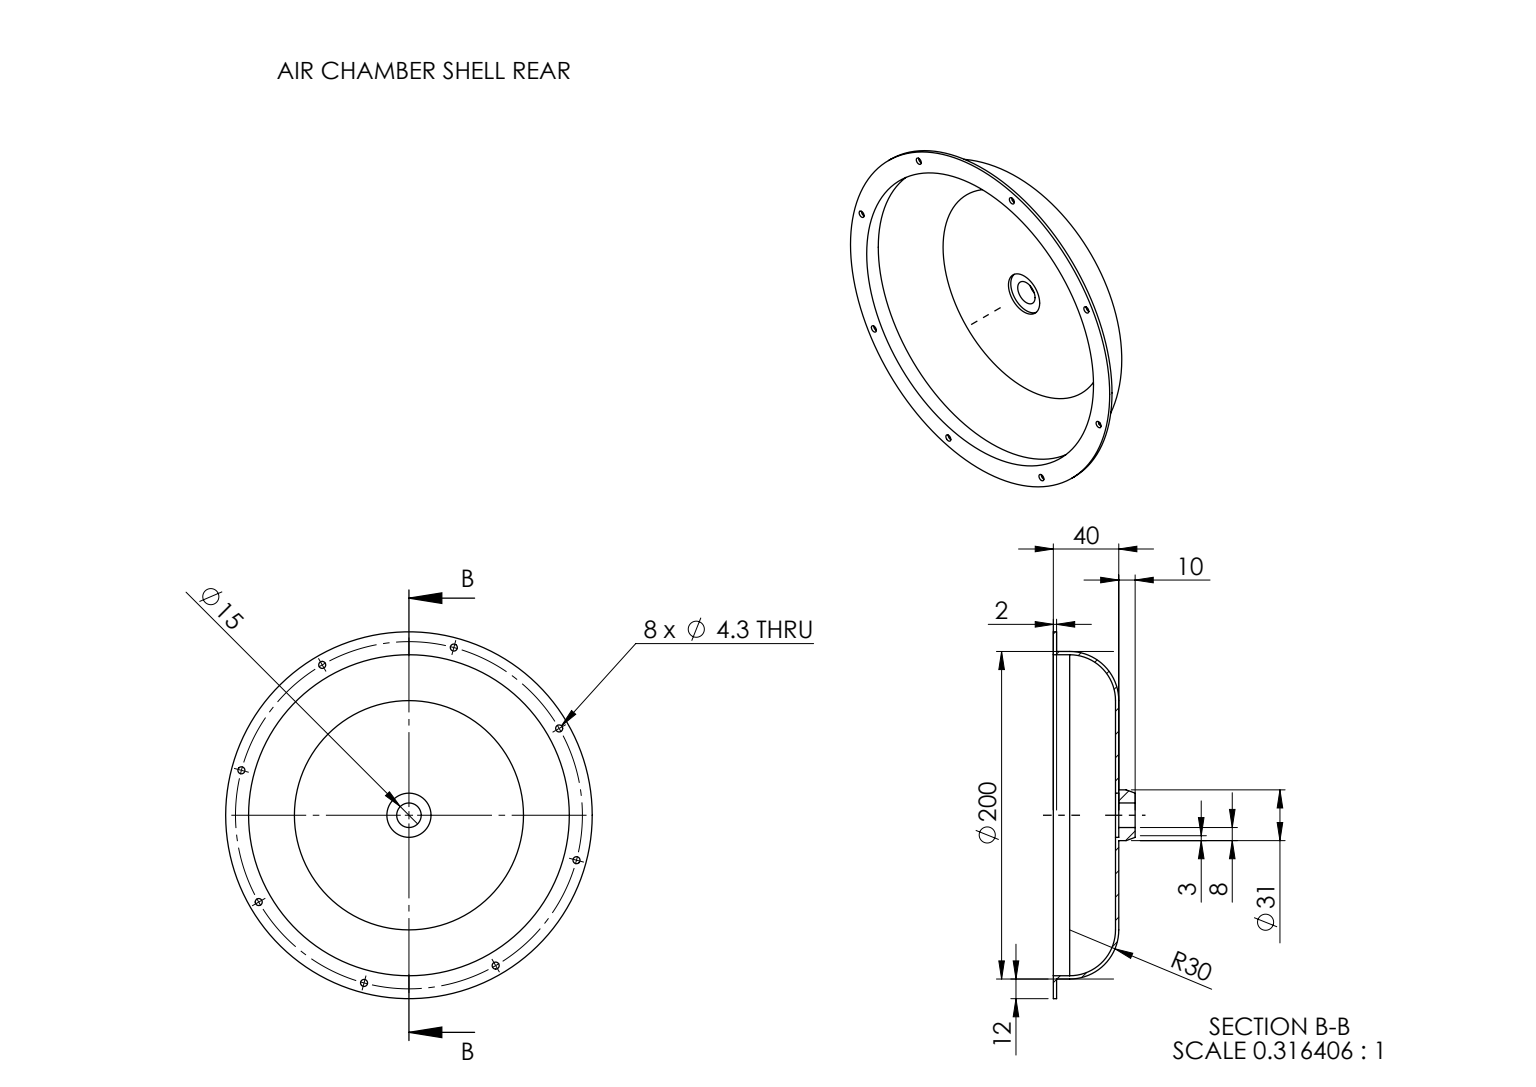
ISO-10303-21;
HEADER;
FILE_DESCRIPTION (('STEP AP214'),
    '1' );
FILE_NAME ('air chamber shell rear.step',
    '2026-10-08T07:58:12',
    ( '' ),
    ( '' ),
    'SwSTEP 2.0',
    'SolidWorks 2026',
    '' );
FILE_SCHEMA (( 'AUTOMOTIVE_DESIGN' ));
ENDSEC;

DATA;
#7=DIRECTION ( 'NONE',  ( 0.000000000000000000, 0.000000000000000000, -1.000000000000000000 ) ) ;
#68=ORIENTED_EDGE ( 'NONE', *, *, #26579, .F. ) ;
#75=AXIS2_PLACEMENT_3D ( 'NONE', #16121, #13402, #469 ) ;
#77=DIRECTION ( 'NONE',  ( -1.000000000000000000, -0.000000000000000000, -0.000000000000000000 ) ) ;
#93=PLANE ( 'NONE',  #4285 ) ;
#101=CIRCLE ( 'NONE', #26212, 13.50000000000001066 ) ;
#171=VERTEX_POINT ( 'NONE', #1955 ) ;
#187=CARTESIAN_POINT ( 'NONE',  ( 107.5000000000000000, 155.0000000000000000, -6.938893903907228378E-15 ) ) ;
#191=EDGE_CURVE ( 'NONE', #26009, #2264, #14724, .T. ) ;
#230=DIRECTION ( 'NONE',  ( 1.000000000000000000, 0.000000000000000000, 0.000000000000000000 ) ) ;
#283=ORIENTED_EDGE ( 'NONE', *, *, #23034, .T. ) ;
#304=CARTESIAN_POINT ( 'NONE',  ( 115.4999999999999858, 207.9999999999998010, -91.79869280115066488 ) ) ;
#307=FACE_BOUND ( 'NONE', #22866, .T. ) ;
#349=AXIS2_PLACEMENT_3D ( 'NONE', #10435, #20806, #13142 ) ;
#414=ORIENTED_EDGE ( 'NONE', *, *, #20724, .T. ) ;
#434=EDGE_CURVE ( 'NONE', #32282, #27762, #17038, .T. ) ;
#438=ORIENTED_EDGE ( 'NONE', *, *, #191, .T. ) ;
#454=ORIENTED_EDGE ( 'NONE', *, *, #17916, .T. ) ;
#462=SURFACE_STYLE_USAGE ( .BOTH. , #25511 ) ;
#469=DIRECTION ( 'NONE',  ( 0.000000000000000000, 0.000000000000000000, -1.000000000000000000 ) ) ;
#492=CONICAL_SURFACE ( 'NONE', #30975, 15.50000000000001066, 0.3490658503988691153 ) ;
#506=( LENGTH_UNIT ( ) NAMED_UNIT ( * ) SI_UNIT ( .MILLI., .METRE. ) );
#529=ORIENTED_EDGE ( 'NONE', *, *, #7683, .F. ) ;
#536=VERTEX_POINT ( 'NONE', #28106 ) ;
#540=ORIENTED_EDGE ( 'NONE', *, *, #17503, .F. ) ;
#598=EDGE_CURVE ( 'NONE', #2264, #27762, #4180, .T. ) ;
#600=CARTESIAN_POINT ( 'NONE',  ( 115.4999999999999858, 155.0000000000000000, -6.938893903907228378E-15 ) ) ;
#625=DIRECTION ( 'NONE',  ( 0.000000000000000000, 0.000000000000000000, -1.000000000000000000 ) ) ;
#670=PRODUCT_CONTEXT ( 'NONE', #3757, 'mechanical' ) ;
#673=CONICAL_SURFACE ( 'NONE', #14801, 15.50000000000001066, 0.3490658503988691153 ) ;
#713=FACE_OUTER_BOUND ( 'NONE', #1487, .T. ) ;
#776=CIRCLE ( 'NONE', #1871, 69.99999999999998579 ) ;
#832=SURFACE_STYLE_FILL_AREA ( #18565 ) ;
#833=DIRECTION ( 'NONE',  ( 0.000000000000000000, 0.000000000000000000, -1.000000000000000000 ) ) ;
#862=ORIENTED_EDGE ( 'NONE', *, *, #26257, .T. ) ;
#903=PRODUCT_DEFINITION_CONTEXT ( 'detailed design', #2680, 'design' ) ;
#950=CIRCLE ( 'NONE', #16649, 27.99999999999999645 ) ;
#961=CARTESIAN_POINT ( 'NONE',  ( 117.5000000000000000, 63.20130719884917170, -52.99999999999946709 ) ) ;
#971=AXIS2_PLACEMENT_3D ( 'NONE', #10766, #21306, #3410 ) ;
#1073=EDGE_LOOP ( 'NONE', ( #10094, #23123, #12443, #529 ) ) ;
#1133=FACE_OUTER_BOUND ( 'NONE', #17035, .T. ) ;
#1157=DIRECTION ( 'NONE',  ( 0.000000000000000000, 0.000000000000000000, -1.000000000000000000 ) ) ;
#1188=ORIENTED_EDGE ( 'NONE', *, *, #27275, .F. ) ;
#1230=CARTESIAN_POINT ( 'NONE',  ( 115.4999999999999858, 51.09158283380785548, 28.95509836041905771 ) ) ;
#1232=MANIFOLD_SOLID_BREP ( 'CirPattern1', #28098 ) ;
#1268=ORIENTED_EDGE ( 'NONE', *, *, #4948, .F. ) ;
#1283=ORIENTED_EDGE ( 'NONE', *, *, #598, .T. ) ;
#1365=EDGE_LOOP ( 'NONE', ( #22857, #1283 ) ) ;
#1371=EDGE_CURVE ( 'NONE', #3136, #6813, #17831, .T. ) ;
#1414=DIRECTION ( 'NONE',  ( 0.000000000000000000, 0.000000000000000000, -1.000000000000000000 ) ) ;
#1450=EDGE_LOOP ( 'NONE', ( #15818, #25203 ) ) ;
#1487=EDGE_LOOP ( 'NONE', ( #7285, #14189, #23041, #24412 ) ) ;
#1501=DIRECTION ( 'NONE',  ( 0.000000000000000000, 1.000000000000000000, -9.682177540335733218E-15 ) ) ;
#1530=CIRCLE ( 'NONE', #18391, 112.0000000000000426 ) ;
#1665=DIRECTION ( 'NONE',  ( 1.000000000000000000, 0.000000000000000000, 0.000000000000000000 ) ) ;
#1738=EDGE_LOOP ( 'NONE', ( #5719, #22132, #19511, #15323 ) ) ;
#1752=DIRECTION ( 'NONE',  ( 0.000000000000000000, -0.7071067811865434649, 0.7071067811865515695 ) ) ;
#1760=DIRECTION ( 'NONE',  ( -1.000000000000000000, 0.000000000000000000, -0.000000000000000000 ) ) ;
#1788=AXIS2_PLACEMENT_3D ( 'NONE', #23905, #3451, #6004 ) ;
#1798=ADVANCED_FACE ( 'NONE', ( #23430, #1969 ), #93, .T. ) ;
#1801=CARTESIAN_POINT ( 'NONE',  ( 117.5000000000000000, 61.05130719884917312, -52.99999999999945999 ) ) ;
#1817=CIRCLE ( 'NONE', #3443, 69.99999999999998579 ) ;
#1831=CARTESIAN_POINT ( 'NONE',  ( 115.4999999999999858, 102.0000000000001990, 91.79869280115065067 ) ) ;
#1852=DIRECTION ( 'NONE',  ( 1.000000000000000000, 0.000000000000000000, 0.000000000000000000 ) ) ;
#1862=ORIENTED_EDGE ( 'NONE', *, *, #7924, .F. ) ;
#1871=AXIS2_PLACEMENT_3D ( 'NONE', #22106, #6777, #17162 ) ;
#1916=VERTEX_POINT ( 'NONE', #11603 ) ;
#1943=DIRECTION ( 'NONE',  ( 0.000000000000000000, 0.000000000000000000, -1.000000000000000000 ) ) ;
#1955=CARTESIAN_POINT ( 'NONE',  ( 77.50000000000000000, 155.0000000000000000, -15.50000000000001776 ) ) ;
#1969=FACE_OUTER_BOUND ( 'NONE', #1365, .T. ) ;
#1973=VECTOR ( 'NONE', #1760, 1000.000000000000000 ) ;
#2026=AXIS2_PLACEMENT_3D ( 'NONE', #600, #24260, #8937 ) ;
#2045=VERTEX_POINT ( 'NONE', #8540 ) ;
#2054=ORIENTED_EDGE ( 'NONE', *, *, #8945, .T. ) ;
#2077=EDGE_LOOP ( 'NONE', ( #31532, #20694 ) ) ;
#2145=DIRECTION ( 'NONE',  ( -1.000000000000000000, 0.000000000000000000, 0.000000000000000000 ) ) ;
#2183=CYLINDRICAL_SURFACE ( 'NONE', #10236, 2.149999999999996803 ) ;
#2198=FACE_BOUND ( 'NONE', #2251, .T. ) ;
#2234=DIRECTION ( 'NONE',  ( 0.000000000000000000, 0.000000000000000000, -1.000000000000000000 ) ) ;
#2251=EDGE_LOOP ( 'NONE', ( #26956, #17710 ) ) ;
#2264=VERTEX_POINT ( 'NONE', #4435 ) ;
#2283=DIRECTION ( 'NONE',  ( 0.000000000000000000, -0.7071067811865540120, -0.7071067811865411334 ) ) ;
#2287=EDGE_CURVE ( 'NONE', #30017, #18599, #30683, .T. ) ;
#2336=CARTESIAN_POINT ( 'NONE',  ( 115.4999999999999858, 207.9999999999998010, -91.79869280115066488 ) ) ;
#2340=CIRCLE ( 'NONE', #6134, 98.00000000000000000 ) ;
#2351=EDGE_LOOP ( 'NONE', ( #6560, #11998 ) ) ;
#2383=AXIS2_PLACEMENT_3D ( 'NONE', #5252, #30654, #20597 ) ;
#2385=ORIENTED_EDGE ( 'NONE', *, *, #25125, .T. ) ;
#2404=AXIS2_PLACEMENT_3D ( 'NONE', #8872, #11941, #4266 ) ;
#2451=DIRECTION ( 'NONE',  ( 0.000000000000000000, 0.7071067811865475727, 0.7071067811865475727 ) ) ;
#2472=ORIENTED_EDGE ( 'NONE', *, *, #5437, .T. ) ;
#2481=CYLINDRICAL_SURFACE ( 'NONE', #11610, 2.149999999999999023 ) ;
#2516=ADVANCED_FACE ( 'NONE', ( #25896 ), #18566, .F. ) ;
#2537=FACE_BOUND ( 'NONE', #23999, .T. ) ;
#2601=FACE_OUTER_BOUND ( 'NONE', #15989, .T. ) ;
#2624=EDGE_CURVE ( 'NONE', #33027, #13306, #29875, .T. ) ;
#2637=DIRECTION ( 'NONE',  ( -1.000000000000000000, 0.000000000000000000, 0.000000000000000000 ) ) ;
#2680=APPLICATION_CONTEXT ( 'automotive_design' ) ;
#2681=AXIS2_PLACEMENT_3D ( 'NONE', #20295, #24901, #6678 ) ;
#2686=DIRECTION ( 'NONE',  ( -1.000000000000000000, -0.000000000000000000, -0.000000000000000000 ) ) ;
#2733=ORIENTED_EDGE ( 'NONE', *, *, #21234, .T. ) ;
#2774=AXIS2_PLACEMENT_3D ( 'NONE', #31193, #5458, #4959 ) ;
#2784=CARTESIAN_POINT ( 'NONE',  ( 79.50000000000000000, 155.0000000000000000, -69.99999999999998579 ) ) ;
#2786=FACE_BOUND ( 'NONE', #10971, .T. ) ;
#2808=ADVANCED_FACE ( 'NONE', ( #9001 ), #25061, .T. ) ;
#2811=EDGE_LOOP ( 'NONE', ( #20272, #1188, #20856, #9872 ) ) ;
#2863=CARTESIAN_POINT ( 'NONE',  ( 72.99495483890930814, 155.0000000000000000, -15.50000000000001776 ) ) ;
#2891=TOROIDAL_SURFACE ( 'NONE', #19225, 69.99999999999998579, 27.99999999999999645 ) ;
#2907=LINE ( 'NONE', #21126, #5343 ) ;
#2914=CARTESIAN_POINT ( 'NONE',  ( 115.4999999999999858, 51.09158283380784837, 28.95509836041906482 ) ) ;
#2953=CIRCLE ( 'NONE', #13273, 2.149999999999999023 ) ;
#3007=ORIENTED_EDGE ( 'NONE', *, *, #21235, .T. ) ;
#3010=DIRECTION ( 'NONE',  ( -1.000000000000000000, -0.000000000000000000, -0.000000000000000000 ) ) ;
#3081=EDGE_LOOP ( 'NONE', ( #11713, #8377, #3706, #13143 ) ) ;
#3082=EDGE_CURVE ( 'NONE', #10769, #27181, #18017, .T. ) ;
#3128=AXIS2_PLACEMENT_3D ( 'NONE', #20706, #25988, #29042 ) ;
#3136=VERTEX_POINT ( 'NONE', #33006 ) ;
#3150=DIRECTION ( 'NONE',  ( 1.000000000000000000, -0.000000000000000000, -0.000000000000000000 ) ) ;
#3162=AXIS2_PLACEMENT_3D ( 'NONE', #6462, #4579, #19574 ) ;
#3166=ORIENTED_EDGE ( 'NONE', *, *, #26579, .T. ) ;
#3182=AXIS2_PLACEMENT_3D ( 'NONE', #6530, #30205, #32410 ) ;
#3227=CARTESIAN_POINT ( 'NONE',  ( 115.4999999999999858, 126.0449016395812691, -103.9084171661922369 ) ) ;
#3230=VECTOR ( 'NONE', #6116, 1000.000000000000000 ) ;
#3252=EDGE_CURVE ( 'NONE', #5646, #15657, #33360, .T. ) ;
#3280=DIRECTION ( 'NONE',  ( -1.000000000000000000, 0.000000000000000000, -0.000000000000000000 ) ) ;
#3299=FACE_OUTER_BOUND ( 'NONE', #22987, .T. ) ;
#3328=EDGE_LOOP ( 'NONE', ( #4132, #17295 ) ) ;
#3354=ADVANCED_FACE ( 'NONE', ( #10372 ), #10201, .F. ) ;
#3410=DIRECTION ( 'NONE',  ( 0.000000000000000000, 0.000000000000000000, -1.000000000000000000 ) ) ;
#3433=CARTESIAN_POINT ( 'NONE',  ( 117.5000000000000000, 155.0000000000000000, -6.938893903907228378E-15 ) ) ;
#3443=AXIS2_PLACEMENT_3D ( 'NONE', #27976, #32741, #17244 ) ;
#3451=DIRECTION ( 'NONE',  ( 1.000000000000000000, 0.000000000000000000, 0.000000000000000000 ) ) ;
#3478=ORIENTED_EDGE ( 'NONE', *, *, #28138, .F. ) ;
#3558=SHAPE_DEFINITION_REPRESENTATION ( #12711, #19592 ) ;
#3599=CIRCLE ( 'NONE', #21614, 97.99999999999997158 ) ;
#3706=ORIENTED_EDGE ( 'NONE', *, *, #7107, .T. ) ;
#3709=EDGE_CURVE ( 'NONE', #5646, #31059, #20736, .T. ) ;
#3737=EDGE_CURVE ( 'NONE', #7925, #10430, #29432, .T. ) ;
#3757=APPLICATION_CONTEXT ( 'automotive_design' ) ;
#3823=VERTEX_POINT ( 'NONE', #30731 ) ;
#3850=CARTESIAN_POINT ( 'NONE',  ( 77.50000000000000000, 155.0000000000000000, -6.938893903907228378E-15 ) ) ;
#3894=EDGE_CURVE ( 'NONE', #10681, #3823, #25105, .T. ) ;
#3937=CARTESIAN_POINT ( 'NONE',  ( 115.4999999999999858, 155.0000000000000000, -6.938893903907228378E-15 ) ) ;
#3983=AXIS2_PLACEMENT_3D ( 'NONE', #32618, #27001, #19510 ) ;
#3984=CARTESIAN_POINT ( 'NONE',  ( 107.5000000000000000, 155.0000000000000000, 69.99999999999998579 ) ) ;
#4000=DIRECTION ( 'NONE',  ( 0.000000000000000000, -0.7071067811865346942, 0.7071067811865604513 ) ) ;
#4008=TOROIDAL_SURFACE ( 'NONE', #10009, 69.99999999999998579, 30.00000000000000000 ) ;
#4047=PLANE ( 'NONE',  #27123 ) ;
#4125=EDGE_LOOP ( 'NONE', ( #33172, #32411, #16064, #3478 ) ) ;
#4132=ORIENTED_EDGE ( 'NONE', *, *, #27275, .T. ) ;
#4180=CIRCLE ( 'NONE', #15058, 13.50000000000001066 ) ;
#4206=EDGE_LOOP ( 'NONE', ( #540, #18309 ) ) ;
#4221=AXIS2_PLACEMENT_3D ( 'NONE', #8999, #1665, #1501 ) ;
#4252=EDGE_CURVE ( 'NONE', #3823, #10681, #19124, .T. ) ;
#4266=DIRECTION ( 'NONE',  ( 1.000000000000000000, 0.000000000000000000, 0.000000000000000000 ) ) ;
#4285=AXIS2_PLACEMENT_3D ( 'NONE', #15423, #12866, #28550 ) ;
#4289=ORIENTED_EDGE ( 'NONE', *, *, #29372, .F. ) ;
#4300=CARTESIAN_POINT ( 'NONE',  ( 115.4999999999999858, 52.61186241335891367, 27.43481878086798176 ) ) ;
#4331=AXIS2_PLACEMENT_3D ( 'NONE', #18954, #26951, #10796 ) ;
#4332=ADVANCED_FACE ( 'NONE', ( #6323 ), #29500, .F. ) ;
#4349=VERTEX_POINT ( 'NONE', #27117 ) ;
#4352=CARTESIAN_POINT ( 'NONE',  ( 77.50000000000000000, 155.0000000000000000, 69.99999999999998579 ) ) ;
#4362=DIRECTION ( 'NONE',  ( 0.000000000000000000, 0.000000000000000000, 1.000000000000000000 ) ) ;
#4398=EDGE_CURVE ( 'NONE', #171, #13101, #11448, .T. ) ;
#4411=CARTESIAN_POINT ( 'NONE',  ( 115.4999999999999858, 244.6486928011512134, 52.99999999999884892 ) ) ;
#4426=EDGE_LOOP ( 'NONE', ( #26831, #11930, #30542, #23954 ) ) ;
#4435=CARTESIAN_POINT ( 'NONE',  ( 77.50000000000000000, 155.0000000000000000, -13.50000000000001776 ) ) ;
#4490=EDGE_CURVE ( 'NONE', #1916, #18599, #24575, .T. ) ;
#4499=LINE ( 'NONE', #28006, #21896 ) ;
#4514=CARTESIAN_POINT ( 'NONE',  ( 117.5000000000000000, 207.9999999999998010, -89.64869280115065919 ) ) ;
#4548=AXIS2_PLACEMENT_3D ( 'NONE', #31582, #8247, #11798 ) ;
#4566=ORIENTED_EDGE ( 'NONE', *, *, #8901, .F. ) ;
#4579=DIRECTION ( 'NONE',  ( 1.000000000000000000, 0.000000000000000000, 0.000000000000000000 ) ) ;
#4586=COLOUR_RGB ( '', 0.72549020, 0.75294118, 0.79215686) ;
#4604=CARTESIAN_POINT ( 'NONE',  ( 117.5000000000000000, 244.6486928011512134, 52.99999999999884892 ) ) ;
#4637=DIRECTION ( 'NONE',  ( 0.000000000000000000, 0.000000000000000000, -1.000000000000000000 ) ) ;
#4646=DIRECTION ( 'NONE',  ( 1.000000000000000000, 0.000000000000000000, 0.000000000000000000 ) ) ;
#4649=ORIENTED_EDGE ( 'NONE', *, *, #2624, .T. ) ;
#4688=CARTESIAN_POINT ( 'NONE',  ( 72.99495483890930814, 155.0000000000000000, -6.938893903907228378E-15 ) ) ;
#4690=CARTESIAN_POINT ( 'NONE',  ( 115.4999999999999858, 258.9084171661918958, -28.95509836041981444 ) ) ;
#4719=EDGE_CURVE ( 'NONE', #27181, #10769, #22400, .T. ) ;
#4762=ORIENTED_EDGE ( 'NONE', *, *, #17424, .T. ) ;
#4797=CIRCLE ( 'NONE', #3162, 112.0000000000000426 ) ;
#4802=ORIENTED_EDGE ( 'NONE', *, *, #598, .F. ) ;
#4822=DIRECTION ( 'NONE',  ( -1.000000000000000000, 0.000000000000000000, 0.000000000000000000 ) ) ;
#4862=LINE ( 'NONE', #28374, #29556 ) ;
#4902=ORIENTED_EDGE ( 'NONE', *, *, #19173, .F. ) ;
#4930=ORIENTED_EDGE ( 'NONE', *, *, #12672, .F. ) ;
#4948=EDGE_CURVE ( 'NONE', #22445, #13672, #13175, .T. ) ;
#4959=DIRECTION ( 'NONE',  ( 0.000000000000000000, 0.7071067811865442421, -0.7071067811865506814 ) ) ;
#4964=EDGE_CURVE ( 'NONE', #19918, #8949, #23184, .T. ) ;
#5016=ORIENTED_EDGE ( 'NONE', *, *, #29173, .F. ) ;
#5019=EDGE_CURVE ( 'NONE', #25798, #12782, #19635, .T. ) ;
#5023=EDGE_CURVE ( 'NONE', #18870, #7638, #28873, .T. ) ;
#5080=AXIS2_PLACEMENT_3D ( 'NONE', #23053, #4822, #22367 ) ;
#5102=ORIENTED_EDGE ( 'NONE', *, *, #28904, .T. ) ;
#5113=ORIENTED_EDGE ( 'NONE', *, *, #8496, .F. ) ;
#5136=ORIENTED_EDGE ( 'NONE', *, *, #19362, .F. ) ;
#5252=CARTESIAN_POINT ( 'NONE',  ( 117.5000000000000000, 127.5651812191323557, -102.3881375866411645 ) ) ;
#5279=CARTESIAN_POINT ( 'NONE',  ( 121.3406204335659879, 155.0000000000000000, -6.938893903907228378E-15 ) ) ;
#5303=DIRECTION ( 'NONE',  ( 0.9396926207859072067, 4.188538737677028743E-17, 0.3420201433256717105 ) ) ;
#5338=DIRECTION ( 'NONE',  ( -1.000000000000000000, 0.000000000000000000, 0.000000000000000000 ) ) ;
#5343=VECTOR ( 'NONE', #26085, 1000.000000000000000 ) ;
#5347=DIRECTION ( 'NONE',  ( -1.000000000000000000, -0.000000000000000000, 0.000000000000000000 ) ) ;
#5397=ORIENTED_EDGE ( 'NONE', *, *, #4252, .T. ) ;
#5437=EDGE_CURVE ( 'NONE', #10401, #5683, #4797, .T. ) ;
#5458=DIRECTION ( 'NONE',  ( -1.000000000000000000, 0.000000000000000000, 0.000000000000000000 ) ) ;
#5473=LINE ( 'NONE', #31537, #24283 ) ;
#5525=VECTOR ( 'NONE', #13656, 1000.000000000000000 ) ;
#5639=AXIS2_PLACEMENT_3D ( 'NONE', #31026, #25731, #28461 ) ;
#5646=VERTEX_POINT ( 'NONE', #4514 ) ;
#5670=DIRECTION ( 'NONE',  ( -1.000000000000000000, -0.000000000000000000, -0.000000000000000000 ) ) ;
#5683=VERTEX_POINT ( 'NONE', #22575 ) ;
#5719=ORIENTED_EDGE ( 'NONE', *, *, #3737, .F. ) ;
#5725=( NAMED_UNIT ( * ) PLANE_ANGLE_UNIT ( ) SI_UNIT ( $, .RADIAN. ) );
#5781=CARTESIAN_POINT ( 'NONE',  ( 79.50000000000000000, 155.0000000000000000, 13.50000000000000355 ) ) ;
#5787=DIRECTION ( 'NONE',  ( 0.000000000000000000, -1.000000000000000000, 9.682177540335733218E-15 ) ) ;
#5843=ORIENTED_EDGE ( 'NONE', *, *, #21234, .F. ) ;
#5862=DIRECTION ( 'NONE',  ( 0.000000000000000000, 1.000000000000000000, -3.227392513445223895E-15 ) ) ;
#5868=CYLINDRICAL_SURFACE ( 'NONE', #2026, 112.0000000000000426 ) ;
#5869=VERTEX_POINT ( 'NONE', #7927 ) ;
#5916=DIRECTION ( 'NONE',  ( 0.000000000000000000, -0.7071067811865540120, -0.7071067811865411334 ) ) ;
#5926=FACE_OUTER_BOUND ( 'NONE', #26057, .T. ) ;
#5953=EDGE_CURVE ( 'NONE', #21331, #2045, #25465, .T. ) ;
#5962=ORIENTED_EDGE ( 'NONE', *, *, #10995, .T. ) ;
#5965=ORIENTED_EDGE ( 'NONE', *, *, #20724, .F. ) ;
#6004=DIRECTION ( 'NONE',  ( 0.000000000000000000, 0.000000000000000000, -1.000000000000000000 ) ) ;
#6026=CARTESIAN_POINT ( 'NONE',  ( 115.4999999999999858, 63.20130719884917170, -52.99999999999946709 ) ) ;
#6031=EDGE_CURVE ( 'NONE', #20901, #28279, #1530, .T. ) ;
#6095=( NAMED_UNIT ( * ) PLANE_ANGLE_UNIT ( ) SI_UNIT ( $, .RADIAN. ) );
#6116=DIRECTION ( 'NONE',  ( -1.000000000000000000, 0.000000000000000000, 0.000000000000000000 ) ) ;
#6134=AXIS2_PLACEMENT_3D ( 'NONE', #9099, #7064, #25108 ) ;
#6139=AXIS2_PLACEMENT_3D ( 'NONE', #21230, #9074, #31625 ) ;
#6143=FACE_OUTER_BOUND ( 'NONE', #15317, .T. ) ;
#6154=DIRECTION ( 'NONE',  ( 0.000000000000000000, 0.000000000000000000, 1.000000000000000000 ) ) ;
#6178=AXIS2_PLACEMENT_3D ( 'NONE', #13035, #31270, #7931 ) ;
#6200=CYLINDRICAL_SURFACE ( 'NONE', #16792, 2.149999999999999023 ) ;
#6215=AXIS2_PLACEMENT_3D ( 'NONE', #31991, #19049, #29438 ) ;
#6217=ORIENTED_EDGE ( 'NONE', *, *, #19362, .T. ) ;
#6245=ADVANCED_FACE ( 'NONE', ( #22193 ), #32582, .F. ) ;
#6270=CARTESIAN_POINT ( 'NONE',  ( 117.5000000000000000, 127.5651812191323557, -102.3881375866411645 ) ) ;
#6319=CIRCLE ( 'NONE', #17271, 2.149999999999985256 ) ;
#6323=FACE_OUTER_BOUND ( 'NONE', #3081, .T. ) ;
#6365=DIRECTION ( 'NONE',  ( 0.000000000000000000, 0.000000000000000000, 1.000000000000000000 ) ) ;
#6462=CARTESIAN_POINT ( 'NONE',  ( 115.4999999999999858, 155.0000000000000000, -6.938893903907228378E-15 ) ) ;
#6530=CARTESIAN_POINT ( 'NONE',  ( 115.4999999999999858, 52.61186241335891367, 27.43481878086798176 ) ) ;
#6531=ORIENTED_EDGE ( 'NONE', *, *, #191, .F. ) ;
#6560=ORIENTED_EDGE ( 'NONE', *, *, #28904, .F. ) ;
#6567=ORIENTED_EDGE ( 'NONE', *, *, #17503, .T. ) ;
#6580=CARTESIAN_POINT ( 'NONE',  ( 77.50000000000000000, 155.0000000000000000, 15.50000000000000355 ) ) ;
#6592=ADVANCED_FACE ( 'NONE', ( #1133 ), #16798, .F. ) ;
#6621=AXIS2_PLACEMENT_3D ( 'NONE', #3433, #29167, #6154 ) ;
#6657=CARTESIAN_POINT ( 'NONE',  ( 115.4999999999999858, 102.0000000000001990, 89.64869280115064498 ) ) ;
#6678=DIRECTION ( 'NONE',  ( 0.000000000000000000, 0.000000000000000000, -1.000000000000000000 ) ) ;
#6770=MECHANICAL_DESIGN_GEOMETRIC_PRESENTATION_REPRESENTATION('',(#8929),#12761);
#6774=VERTEX_POINT ( 'NONE', #15086 ) ;
#6777=DIRECTION ( 'NONE',  ( -1.000000000000000000, -0.000000000000000000, -0.000000000000000000 ) ) ;
#6813=VERTEX_POINT ( 'NONE', #1801 ) ;
#6831=CYLINDRICAL_SURFACE ( 'NONE', #23613, 7.500000000000015099 ) ;
#6885=DIRECTION ( 'NONE',  ( 0.000000000000000000, 1.000000000000000000, -3.227392513445244800E-15 ) ) ;
#6892=CARTESIAN_POINT ( 'NONE',  ( 117.5000000000000000, 155.0000000000000000, -6.938893903907228378E-15 ) ) ;
#6902=VERTEX_POINT ( 'NONE', #28383 ) ;
#6919=CARTESIAN_POINT ( 'NONE',  ( 72.99495483890930814, 155.0000000000000000, -6.938893903907228378E-15 ) ) ;
#6935=DIRECTION ( 'NONE',  ( 0.000000000000000000, 0.000000000000000000, 1.000000000000000000 ) ) ;
#6984=ORIENTED_EDGE ( 'NONE', *, *, #27838, .F. ) ;
#7024=TOROIDAL_SURFACE ( 'NONE', #2681, 69.99999999999998579, 27.99999999999999645 ) ;
#7064=DIRECTION ( 'NONE',  ( 1.000000000000000000, 0.000000000000000000, 0.000000000000000000 ) ) ;
#7072=DIRECTION ( 'NONE',  ( -1.000000000000000000, -0.000000000000000000, -0.000000000000000000 ) ) ;
#7107=EDGE_CURVE ( 'NONE', #16763, #31655, #26322, .T. ) ;
#7142=DIRECTION ( 'NONE',  ( -1.000000000000000000, -0.000000000000000000, -0.000000000000000000 ) ) ;
#7145=AXIS2_PLACEMENT_3D ( 'NONE', #18693, #16919, #15797 ) ;
#7160=CARTESIAN_POINT ( 'NONE',  ( 77.50000000000000000, 155.0000000000000000, 13.50000000000000355 ) ) ;
#7166=AXIS2_PLACEMENT_3D ( 'NONE', #33449, #10120, #2451 ) ;
#7190=ADVANCED_FACE ( 'NONE', ( #21870 ), #6200, .F. ) ;
#7200=CIRCLE ( 'NONE', #20254, 2.149999999999999023 ) ;
#7254=ADVANCED_FACE ( 'NONE', ( #29711 ), #492, .T. ) ;
#7285=ORIENTED_EDGE ( 'NONE', *, *, #15353, .F. ) ;
#7302=CARTESIAN_POINT ( 'NONE',  ( 115.4999999999999858, 52.61186241335891367, 27.43481878086798176 ) ) ;
#7317=FACE_BOUND ( 'NONE', #15067, .T. ) ;
#7338=ORIENTED_EDGE ( 'NONE', *, *, #3709, .T. ) ;
#7340=DIRECTION ( 'NONE',  ( -1.000000000000000000, -0.000000000000000000, -0.000000000000000000 ) ) ;
#7406=LINE ( 'NONE', #12847, #17581 ) ;
#7427=ADVANCED_FACE ( 'NONE', ( #9782 ), #32429, .F. ) ;
#7451=ORIENTED_EDGE ( 'NONE', *, *, #20414, .T. ) ;
#7477=DIRECTION ( 'NONE',  ( 0.000000000000000000, 0.000000000000000000, 1.000000000000000000 ) ) ;
#7481=DIRECTION ( 'NONE',  ( 1.000000000000000000, 0.000000000000000000, 0.000000000000000000 ) ) ;
#7494=EDGE_CURVE ( 'NONE', #30420, #7638, #15710, .T. ) ;
#7540=ADVANCED_FACE ( 'NONE', ( #18123 ), #7738, .F. ) ;
#7545=EDGE_LOOP ( 'NONE', ( #22267, #16346 ) ) ;
#7557=CARTESIAN_POINT ( 'NONE',  ( 117.5000000000000000, 155.0000000000000000, -6.938893903907228378E-15 ) ) ;
#7571=CARTESIAN_POINT ( 'NONE',  ( 117.5000000000000000, 129.0854607986834424, -100.8678580070900921 ) ) ;
#7588=AXIS2_PLACEMENT_3D ( 'NONE', #21114, #33566, #28793 ) ;
#7638=VERTEX_POINT ( 'NONE', #12505 ) ;
#7683=EDGE_CURVE ( 'NONE', #3136, #27139, #31245, .T. ) ;
#7738=CYLINDRICAL_SURFACE ( 'NONE', #32579, 2.149999999999994138 ) ;
#7752=ORIENTED_EDGE ( 'NONE', *, *, #8496, .T. ) ;
#7814=FACE_OUTER_BOUND ( 'NONE', #8127, .T. ) ;
#7831=ORIENTED_EDGE ( 'NONE', *, *, #33511, .F. ) ;
#7869=EDGE_LOOP ( 'NONE', ( #24489, #16038 ) ) ;
#7874=FACE_OUTER_BOUND ( 'NONE', #18824, .T. ) ;
#7890=DIRECTION ( 'NONE',  ( -1.000000000000000000, 0.000000000000000000, -0.000000000000000000 ) ) ;
#7918=ORIENTED_EDGE ( 'NONE', *, *, #26651, .F. ) ;
#7924=EDGE_CURVE ( 'NONE', #4349, #5869, #18470, .T. ) ;
#7925=VERTEX_POINT ( 'NONE', #16556 ) ;
#7927=CARTESIAN_POINT ( 'NONE',  ( 67.50000000000000000, 155.0000000000000000, -13.49999999999997691 ) ) ;
#7931=DIRECTION ( 'NONE',  ( 0.000000000000000000, 0.000000000000000000, 1.000000000000000000 ) ) ;
#7948=CARTESIAN_POINT ( 'NONE',  ( 117.5000000000000000, 51.09158283380784837, 28.95509836041906837 ) ) ;
#7954=EDGE_CURVE ( 'NONE', #9032, #12934, #25540, .T. ) ;
#8046=CIRCLE ( 'NONE', #30327, 2.149999999999985256 ) ;
#8049=CARTESIAN_POINT ( 'NONE',  ( 107.5000000000000000, 155.0000000000000000, -6.938893903907228378E-15 ) ) ;
#8127=EDGE_LOOP ( 'NONE', ( #7338, #30034, #21469, #31896 ) ) ;
#8140=CARTESIAN_POINT ( 'NONE',  ( 117.5000000000000000, 63.20130719884917170, -52.99999999999946709 ) ) ;
#8142=CARTESIAN_POINT ( 'NONE',  ( 115.4999999999999858, 155.0000000000000000, -100.0000000000000000 ) ) ;
#8180=SURFACE_SIDE_STYLE ('',( #832 ) ) ;
#8181=CARTESIAN_POINT ( 'NONE',  ( 115.4999999999999858, 257.3881375866408803, -27.43481878086871717 ) ) ;
#8184=FACE_OUTER_BOUND ( 'NONE', #1738, .T. ) ;
#8247=DIRECTION ( 'NONE',  ( 1.000000000000000000, 0.000000000000000000, 0.000000000000000000 ) ) ;
#8292=DIRECTION ( 'NONE',  ( 0.000000000000000000, 0.000000000000000000, -1.000000000000000000 ) ) ;
#8348=AXIS2_PLACEMENT_3D ( 'NONE', #27979, #4646, #15030 ) ;
#8364=DIRECTION ( 'NONE',  ( -1.000000000000000000, 0.000000000000000000, -0.000000000000000000 ) ) ;
#8377=ORIENTED_EDGE ( 'NONE', *, *, #15569, .T. ) ;
#8390=VECTOR ( 'NONE', #31681, 1000.000000000000000 ) ;
#8489=DIRECTION ( 'NONE',  ( 1.000000000000000000, 0.000000000000000000, 0.000000000000000000 ) ) ;
#8496=EDGE_CURVE ( 'NONE', #9032, #22445, #20970, .T. ) ;
#8540=CARTESIAN_POINT ( 'NONE',  ( 117.5000000000000000, 183.9550983604194698, 103.9084171661920095 ) ) ;
#8559=CARTESIAN_POINT ( 'NONE',  ( 67.50000000000000000, 155.0000000000000000, -6.938893903907228378E-15 ) ) ;
#8610=VECTOR ( 'NONE', #15992, 1000.000000000000114 ) ;
#8616=ORIENTED_EDGE ( 'NONE', *, *, #5953, .F. ) ;
#8619=ORIENTED_EDGE ( 'NONE', *, *, #18971, .T. ) ;
#8630=VECTOR ( 'NONE', #26673, 1000.000000000000000 ) ;
#8634=CARTESIAN_POINT ( 'NONE',  ( 115.4999999999999858, 102.0000000000001990, 91.79869280115065067 ) ) ;
#8635=FACE_OUTER_BOUND ( 'NONE', #19604, .T. ) ;
#8638=DIRECTION ( 'NONE',  ( -1.000000000000000000, -0.000000000000000000, -0.000000000000000000 ) ) ;
#8734=CARTESIAN_POINT ( 'NONE',  ( 115.4999999999999858, 257.3881375866408803, -27.43481878086871717 ) ) ;
#8793=DIRECTION ( 'NONE',  ( 1.000000000000000000, 0.000000000000000000, 0.000000000000000000 ) ) ;
#8872=CARTESIAN_POINT ( 'NONE',  ( 0.000000000000000000, 0.000000000000000000, 0.000000000000000000 ) ) ;
#8877=CYLINDRICAL_SURFACE ( 'NONE', #10544, 2.149999999999994138 ) ;
#8893=AXIS2_PLACEMENT_3D ( 'NONE', #4300, #22532, #15200 ) ;
#8901=EDGE_CURVE ( 'NONE', #5683, #20901, #11916, .T. ) ;
#8926=DIRECTION ( 'NONE',  ( 1.000000000000000000, 0.000000000000000000, 0.000000000000000000 ) ) ;
#8929=STYLED_ITEM ( 'NONE', ( #10899 ), #16530 ) ;
#8937=DIRECTION ( 'NONE',  ( 0.000000000000000000, 0.000000000000000000, -1.000000000000000000 ) ) ;
#8945=EDGE_CURVE ( 'NONE', #14561, #171, #25560, .T. ) ;
#8949=VERTEX_POINT ( 'NONE', #4411 ) ;
#8966=FACE_OUTER_BOUND ( 'NONE', #11004, .T. ) ;
#8999=CARTESIAN_POINT ( 'NONE',  ( 117.5000000000000000, 246.7986928011511907, 52.99999999999882760 ) ) ;
#9001=FACE_OUTER_BOUND ( 'NONE', #10282, .T. ) ;
#9016=ADVANCED_FACE ( 'NONE', ( #26001 ), #20889, .F. ) ;
#9032=VERTEX_POINT ( 'NONE', #7948 ) ;
#9069=CIRCLE ( 'NONE', #28119, 15.50000000000001066 ) ;
#9074=DIRECTION ( 'NONE',  ( 1.000000000000000000, 0.000000000000000000, 0.000000000000000000 ) ) ;
#9091=CARTESIAN_POINT ( 'NONE',  ( 115.4999999999999858, 255.8678580070898363, -25.91453920131762345 ) ) ;
#9099=CARTESIAN_POINT ( 'NONE',  ( 117.5000000000000000, 155.0000000000000000, -6.938893903907228378E-15 ) ) ;
#9100=ADVANCED_FACE ( 'NONE', ( #31929 ), #5868, .T. ) ;
#9112=FACE_BOUND ( 'NONE', #18515, .T. ) ;
#9150=AXIS2_PLACEMENT_3D ( 'NONE', #10047, #7481, #28263 ) ;
#9173=DIRECTION ( 'NONE',  ( -1.000000000000000000, -0.000000000000000000, -0.000000000000000000 ) ) ;
#9201=ORIENTED_EDGE ( 'NONE', *, *, #21789, .T. ) ;
#9240=ORIENTED_EDGE ( 'NONE', *, *, #3082, .F. ) ;
#9299=FACE_OUTER_BOUND ( 'NONE', #15931, .T. ) ;
#9354=VECTOR ( 'NONE', #11527, 1000.000000000000000 ) ;
#9377=AXIS2_PLACEMENT_3D ( 'NONE', #3850, #17137, #12024 ) ;
#9415=CARTESIAN_POINT ( 'NONE',  ( 117.5000000000000000, 180.9145392013172682, 100.8678580070898931 ) ) ;
#9441=DIRECTION ( 'NONE',  ( 0.000000000000000000, -1.000000000000000000, 0.000000000000000000 ) ) ;
#9475=AXIS2_PLACEMENT_3D ( 'NONE', #9845, #25164, #24669 ) ;
#9486=DIRECTION ( 'NONE',  ( 1.000000000000000000, 0.000000000000000000, 0.000000000000000000 ) ) ;
#9487=ORIENTED_EDGE ( 'NONE', *, *, #20414, .F. ) ;
#9497=CYLINDRICAL_SURFACE ( 'NONE', #9475, 2.149999999999985256 ) ;
#9619=FACE_OUTER_BOUND ( 'NONE', #3328, .T. ) ;
#9624=LINE ( 'NONE', #17979, #17251 ) ;
#9636=CYLINDRICAL_SURFACE ( 'NONE', #19709, 13.50000000000001066 ) ;
#9690=UNCERTAINTY_MEASURE_WITH_UNIT (LENGTH_MEASURE( 1.000000000000000082E-05 ), #16325, 'distance_accuracy_value', 'NONE');
#9741=CARTESIAN_POINT ( 'NONE',  ( 77.50000000000000000, 155.0000000000000000, -6.938893903907228378E-15 ) ) ;
#9782=FACE_OUTER_BOUND ( 'NONE', #27679, .T. ) ;
#9792=CARTESIAN_POINT ( 'NONE',  ( 115.4999999999999858, 257.3881375866408803, -27.43481878086871717 ) ) ;
#9845=CARTESIAN_POINT ( 'NONE',  ( 115.4999999999999858, 246.7986928011511907, 52.99999999999882760 ) ) ;
#9872=ORIENTED_EDGE ( 'NONE', *, *, #13553, .F. ) ;
#9930=CIRCLE ( 'NONE', #28438, 2.149999999999985256 ) ;
#9953=CARTESIAN_POINT ( 'NONE',  ( 115.4999999999999858, 182.4348187808683690, 102.3881375866409513 ) ) ;
#9958=CIRCLE ( 'NONE', #16446, 98.00000000000000000 ) ;
#9963=DIRECTION ( 'NONE',  ( 0.000000000000000000, 0.000000000000000000, -1.000000000000000000 ) ) ;
#9965=ORIENTED_EDGE ( 'NONE', *, *, #20838, .F. ) ;
#9977=AXIS2_PLACEMENT_3D ( 'NONE', #28165, #15881, #10946 ) ;
#10009=AXIS2_PLACEMENT_3D ( 'NONE', #8049, #12813, #28984 ) ;
#10023=CIRCLE ( 'NONE', #25229, 97.99999999999997158 ) ;
#10047=CARTESIAN_POINT ( 'NONE',  ( 117.5000000000000000, 155.0000000000000000, -6.938893903907228378E-15 ) ) ;
#10084=CARTESIAN_POINT ( 'NONE',  ( 107.5000000000000000, 155.0000000000000000, -70.00000000000000000 ) ) ;
#10094=ORIENTED_EDGE ( 'NONE', *, *, #1371, .T. ) ;
#10120=DIRECTION ( 'NONE',  ( -1.000000000000000000, -0.000000000000000000, 0.000000000000000000 ) ) ;
#10201=CYLINDRICAL_SURFACE ( 'NONE', #14210, 2.149999999999985256 ) ;
#10236=AXIS2_PLACEMENT_3D ( 'NONE', #7302, #18357, #28247 ) ;
#10282=EDGE_LOOP ( 'NONE', ( #29905, #2385, #12773, #13718 ) ) ;
#10288=FACE_OUTER_BOUND ( 'NONE', #17538, .T. ) ;
#10323=EDGE_CURVE ( 'NONE', #16399, #19918, #14564, .T. ) ;
#10326=DIRECTION ( 'NONE',  ( 0.000000000000000000, 0.000000000000000000, -1.000000000000000000 ) ) ;
#10329=DIRECTION ( 'NONE',  ( 0.000000000000000000, 1.000000000000000000, -3.227392513445223895E-15 ) ) ;
#10369=CARTESIAN_POINT ( 'NONE',  ( 107.5000000000000000, 155.0000000000000000, 97.99999999999997158 ) ) ;
#10372=FACE_OUTER_BOUND ( 'NONE', #20184, .T. ) ;
#10401=VERTEX_POINT ( 'NONE', #32666 ) ;
#10411=DIRECTION ( 'NONE',  ( 0.000000000000000000, 0.000000000000000000, 1.000000000000000000 ) ) ;
#10430=VERTEX_POINT ( 'NONE', #16832 ) ;
#10435=CARTESIAN_POINT ( 'NONE',  ( 79.50000000000000000, 155.0000000000000000, -6.938893903907228378E-15 ) ) ;
#10521=ORIENTED_EDGE ( 'NONE', *, *, #19173, .T. ) ;
#10525=ORIENTED_EDGE ( 'NONE', *, *, #21669, .F. ) ;
#10532=VERTEX_POINT ( 'NONE', #15792 ) ;
#10544=AXIS2_PLACEMENT_3D ( 'NONE', #19274, #11116, #27113 ) ;
#10573=( NAMED_UNIT ( * ) SI_UNIT ( $, .STERADIAN. ) SOLID_ANGLE_UNIT ( ) );
#10618=ADVANCED_FACE ( 'NONE', ( #12568 ), #2183, .F. ) ;
#10622=DIRECTION ( 'NONE',  ( -1.000000000000000000, -0.000000000000000000, -0.000000000000000000 ) ) ;
#10624=DIRECTION ( 'NONE',  ( 0.000000000000000000, 0.000000000000000000, -1.000000000000000000 ) ) ;
#10681=VERTEX_POINT ( 'NONE', #30980 ) ;
#10703=DIRECTION ( 'NONE',  ( -1.000000000000000000, -0.000000000000000000, -0.000000000000000000 ) ) ;
#10757=CARTESIAN_POINT ( 'NONE',  ( 117.5000000000000000, 155.0000000000000000, 98.00000000000000000 ) ) ;
#10766=CARTESIAN_POINT ( 'NONE',  ( 67.50000000000000000, 155.0000000000000000, -6.938893903907228378E-15 ) ) ;
#10769=VERTEX_POINT ( 'NONE', #8142 ) ;
#10795=ORIENTED_EDGE ( 'NONE', *, *, #5019, .F. ) ;
#10796=DIRECTION ( 'NONE',  ( 0.000000000000000000, -0.7071067811865434649, 0.7071067811865515695 ) ) ;
#10847=ADVANCED_FACE ( 'NONE', ( #21072 ), #2891, .F. ) ;
#10899=PRESENTATION_STYLE_ASSIGNMENT (( #28792 ) ) ;
#10946=DIRECTION ( 'NONE',  ( 0.000000000000000000, 0.7071067811865330288, -0.7071067811865621167 ) ) ;
#10965=FACE_OUTER_BOUND ( 'NONE', #20645, .T. ) ;
#10971=EDGE_LOOP ( 'NONE', ( #2054, #15401 ) ) ;
#10985=EDGE_CURVE ( 'NONE', #33564, #10532, #30645, .T. ) ;
#10995=EDGE_CURVE ( 'NONE', #12934, #9032, #16492, .T. ) ;
#11004=EDGE_LOOP ( 'NONE', ( #1862, #28090, #68, #31998 ) ) ;
#11073=CIRCLE ( 'NONE', #8348, 2.149999999999999023 ) ;
#11077=CARTESIAN_POINT ( 'NONE',  ( 67.50000000000000000, 155.0000000000000000, -7.500000000000022204 ) ) ;
#11116=DIRECTION ( 'NONE',  ( -1.000000000000000000, 0.000000000000000000, 0.000000000000000000 ) ) ;
#11180=LINE ( 'NONE', #21557, #8630 ) ;
#11189=EDGE_CURVE ( 'NONE', #31748, #28486, #14873, .T. ) ;
#11204=EDGE_CURVE ( 'NONE', #27181, #18870, #33615, .T. ) ;
#11329=VERTEX_POINT ( 'NONE', #2784 ) ;
#11366=EDGE_CURVE ( 'NONE', #10401, #28279, #18447, .T. ) ;
#11415=CARTESIAN_POINT ( 'NONE',  ( 115.4999999999999858, 155.0000000000000000, -112.0000000000000426 ) ) ;
#11448=LINE ( 'NONE', #32386, #5525 ) ;
#11450=CARTESIAN_POINT ( 'NONE',  ( 115.4999999999999858, 180.9145392013172682, 100.8678580070898931 ) ) ;
#11481=CYLINDRICAL_SURFACE ( 'NONE', #31761, 15.50000000000001066 ) ;
#11488=DIRECTION ( 'NONE',  ( 0.000000000000000000, 0.000000000000000000, 1.000000000000000000 ) ) ;
#11520=CIRCLE ( 'NONE', #25679, 2.149999999999985256 ) ;
#11527=DIRECTION ( 'NONE',  ( -1.000000000000000000, -0.000000000000000000, -0.000000000000000000 ) ) ;
#11603=CARTESIAN_POINT ( 'NONE',  ( 115.4999999999999858, 102.0000000000001990, 93.94869280115062793 ) ) ;
#11610=AXIS2_PLACEMENT_3D ( 'NONE', #33649, #20701, #10329 ) ;
#11628=CIRCLE ( 'NONE', #15974, 2.149999999999994138 ) ;
#11633=ORIENTED_EDGE ( 'NONE', *, *, #14919, .T. ) ;
#11637=ADVANCED_FACE ( 'NONE', ( #713 ), #8877, .F. ) ;
#11658=DIRECTION ( 'NONE',  ( 0.000000000000000000, 1.000000000000000000, -3.227392513445244800E-15 ) ) ;
#11713=ORIENTED_EDGE ( 'NONE', *, *, #31268, .F. ) ;
#11798=DIRECTION ( 'NONE',  ( 0.000000000000000000, 0.000000000000000000, -1.000000000000000000 ) ) ;
#11827=DIRECTION ( 'NONE',  ( -1.000000000000000000, 0.000000000000000000, 0.000000000000000000 ) ) ;
#11831=ADVANCED_FACE ( 'NONE', ( #8184 ), #6831, .F. ) ;
#11894=EDGE_CURVE ( 'NONE', #26009, #32282, #32284, .T. ) ;
#11916=LINE ( 'NONE', #11415, #31545 ) ;
#11930=ORIENTED_EDGE ( 'NONE', *, *, #10323, .T. ) ;
#11941=DIRECTION ( 'NONE',  ( 0.000000000000000000, 0.000000000000000000, 1.000000000000000000 ) ) ;
#11998=ORIENTED_EDGE ( 'NONE', *, *, #5437, .F. ) ;
#12024=DIRECTION ( 'NONE',  ( 0.000000000000000000, 0.000000000000000000, -1.000000000000000000 ) ) ;
#12041=DIRECTION ( 'NONE',  ( 0.000000000000000000, 0.000000000000000000, -1.000000000000000000 ) ) ;
#12051=CARTESIAN_POINT ( 'NONE',  ( 67.50000000000000000, 155.0000000000000000, 7.500000000000007994 ) ) ;
#12165=ORIENTED_EDGE ( 'NONE', *, *, #15906, .T. ) ;
#12222=DIRECTION ( 'NONE',  ( 1.000000000000000000, 0.000000000000000000, 0.000000000000000000 ) ) ;
#12247=DIRECTION ( 'NONE',  ( 1.000000000000000000, 0.000000000000000000, 0.000000000000000000 ) ) ;
#12254=ADVANCED_FACE ( 'NONE', ( #26118, #2786 ), #13166, .F. ) ;
#12335=DIRECTION ( 'NONE',  ( -1.000000000000000000, 0.000000000000000000, 0.000000000000000000 ) ) ;
#12443=ORIENTED_EDGE ( 'NONE', *, *, #15577, .T. ) ;
#12454=DIRECTION ( 'NONE',  ( 0.000000000000000000, 0.000000000000000000, -1.000000000000000000 ) ) ;
#12463=FACE_OUTER_BOUND ( 'NONE', #32654, .T. ) ;
#12505=CARTESIAN_POINT ( 'NONE',  ( 107.5000000000000000, 155.0000000000000000, -100.0000000000000000 ) ) ;
#12561=DIRECTION ( 'NONE',  ( -1.000000000000000000, 0.000000000000000000, 0.000000000000000000 ) ) ;
#12568=FACE_OUTER_BOUND ( 'NONE', #27633, .T. ) ;
#12570=DIRECTION ( 'NONE',  ( -1.000000000000000000, -0.000000000000000000, -0.000000000000000000 ) ) ;
#12642=VECTOR ( 'NONE', #2637, 1000.000000000000000 ) ;
#12671=AXIS2_PLACEMENT_3D ( 'NONE', #8734, #19126, #26785 ) ;
#12672=EDGE_CURVE ( 'NONE', #11329, #17667, #15466, .T. ) ;
#12711=PRODUCT_DEFINITION_SHAPE ( 'NONE', 'NONE',  #27284 ) ;
#12723=EDGE_CURVE ( 'NONE', #24566, #3823, #16010, .T. ) ;
#12761=( GEOMETRIC_REPRESENTATION_CONTEXT ( 3 ) GLOBAL_UNCERTAINTY_ASSIGNED_CONTEXT ( ( #9690 ) ) GLOBAL_UNIT_ASSIGNED_CONTEXT ( ( #16325, #6095, #15833 ) ) REPRESENTATION_CONTEXT ( 'NONE', 'WORKASPACE' ) );
#12773=ORIENTED_EDGE ( 'NONE', *, *, #18971, .F. ) ;
#12782=VERTEX_POINT ( 'NONE', #11077 ) ;
#12813=DIRECTION ( 'NONE',  ( 1.000000000000000000, 0.000000000000000000, 0.000000000000000000 ) ) ;
#12838=ORIENTED_EDGE ( 'NONE', *, *, #6031, .F. ) ;
#12847=CARTESIAN_POINT ( 'NONE',  ( 115.4999999999999858, 129.0854607986834424, -100.8678580070900921 ) ) ;
#12866=DIRECTION ( 'NONE',  ( 1.000000000000000000, 0.000000000000000000, 0.000000000000000000 ) ) ;
#12869=CARTESIAN_POINT ( 'NONE',  ( 115.4999999999999858, 155.0000000000000000, 100.0000000000000000 ) ) ;
#12895=EDGE_LOOP ( 'NONE', ( #5113, #21631, #16611, #10521 ) ) ;
#12920=FACE_BOUND ( 'NONE', #4206, .T. ) ;
#12934=VERTEX_POINT ( 'NONE', #25024 ) ;
#13022=AXIS2_PLACEMENT_3D ( 'NONE', #24945, #9441, #1943 ) ;
#13035=CARTESIAN_POINT ( 'NONE',  ( 117.5000000000000000, 102.0000000000001990, 91.79869280115065067 ) ) ;
#13083=ADVANCED_FACE ( 'NONE', ( #7814 ), #31147, .F. ) ;
#13101=VERTEX_POINT ( 'NONE', #2863 ) ;
#13108=ORIENTED_EDGE ( 'NONE', *, *, #27838, .T. ) ;
#13122=VECTOR ( 'NONE', #12570, 1000.000000000000000 ) ;
#13126=DIRECTION ( 'NONE',  ( 1.000000000000000000, 0.000000000000000000, 0.000000000000000000 ) ) ;
#13142=DIRECTION ( 'NONE',  ( 0.000000000000000000, 0.000000000000000000, -1.000000000000000000 ) ) ;
#13143=ORIENTED_EDGE ( 'NONE', *, *, #21554, .F. ) ;
#13166=PLANE ( 'NONE',  #28511 ) ;
#13169=CARTESIAN_POINT ( 'NONE',  ( 117.5000000000000000, 257.3881375866408803, -27.43481878086871717 ) ) ;
#13175=CIRCLE ( 'NONE', #2774, 2.149999999999984812 ) ;
#13194=PRODUCT_DEFINITION_FORMATION_WITH_SPECIFIED_SOURCE ( 'ANY', '', #17886, .NOT_KNOWN. ) ;
#13273=AXIS2_PLACEMENT_3D ( 'NONE', #23993, #8489, #1157 ) ;
#13290=DIRECTION ( 'NONE',  ( 0.000000000000000000, 0.000000000000000000, 1.000000000000000000 ) ) ;
#13306=VERTEX_POINT ( 'NONE', #30992 ) ;
#13367=ORIENTED_EDGE ( 'NONE', *, *, #5019, .T. ) ;
#13371=FACE_OUTER_BOUND ( 'NONE', #22234, .T. ) ;
#13402=DIRECTION ( 'NONE',  ( -1.000000000000000000, -0.000000000000000000, -0.000000000000000000 ) ) ;
#13434=ORIENTED_EDGE ( 'NONE', *, *, #33465, .T. ) ;
#13469=ADVANCED_FACE ( 'NONE', ( #8635 ), #27025, .F. ) ;
#13484=DIRECTION ( 'NONE',  ( 1.000000000000000000, 0.000000000000000000, 0.000000000000000000 ) ) ;
#13502=EDGE_LOOP ( 'NONE', ( #10795, #32077 ) ) ;
#13514=EDGE_CURVE ( 'NONE', #14561, #20988, #29927, .T. ) ;
#13553=EDGE_CURVE ( 'NONE', #20988, #13101, #28408, .T. ) ;
#13561=CYLINDRICAL_SURFACE ( 'NONE', #32481, 99.99999999999997158 ) ;
#13656=DIRECTION ( 'NONE',  ( -1.000000000000000000, -0.000000000000000000, -0.000000000000000000 ) ) ;
#13672=VERTEX_POINT ( 'NONE', #24643 ) ;
#13684=CARTESIAN_POINT ( 'NONE',  ( 107.5000000000000000, 155.0000000000000000, -6.938893903907228378E-15 ) ) ;
#13718=ORIENTED_EDGE ( 'NONE', *, *, #7494, .F. ) ;
#13757=ORIENTED_EDGE ( 'NONE', *, *, #434, .T. ) ;
#13761=ORIENTED_EDGE ( 'NONE', *, *, #23908, .F. ) ;
#13766=CYLINDRICAL_SURFACE ( 'NONE', #20917, 2.150000000000004352 ) ;
#13773=AXIS2_PLACEMENT_3D ( 'NONE', #22714, #25094, #1752 ) ;
#13810=EDGE_LOOP ( 'NONE', ( #26100, #25461 ) ) ;
#13862=DIRECTION ( 'NONE',  ( 1.000000000000000000, 0.000000000000000000, 0.000000000000000000 ) ) ;
#13870=CARTESIAN_POINT ( 'NONE',  ( 72.99495483890930814, 155.0000000000000000, -6.938893903907228378E-15 ) ) ;
#13939=ORIENTED_EDGE ( 'NONE', *, *, #11189, .F. ) ;
#13962=ORIENTED_EDGE ( 'NONE', *, *, #31210, .T. ) ;
#14063=EDGE_LOOP ( 'NONE', ( #20063, #21006 ) ) ;
#14075=DIRECTION ( 'NONE',  ( 1.000000000000000000, -0.000000000000000000, -0.000000000000000000 ) ) ;
#14145=EDGE_LOOP ( 'NONE', ( #3007, #22219 ) ) ;
#14160=EDGE_CURVE ( 'NONE', #27762, #2264, #101, .T. ) ;
#14189=ORIENTED_EDGE ( 'NONE', *, *, #19529, .T. ) ;
#14205=DIRECTION ( 'NONE',  ( 0.000000000000000000, 1.000000000000000000, -1.224646799147353207E-16 ) ) ;
#14210=AXIS2_PLACEMENT_3D ( 'NONE', #17511, #33192, #20583 ) ;
#14237=AXIS2_PLACEMENT_3D ( 'NONE', #6919, #17310, #14244 ) ;
#14244=DIRECTION ( 'NONE',  ( 0.000000000000000000, 0.000000000000000000, -1.000000000000000000 ) ) ;
#14283=AXIS2_PLACEMENT_3D ( 'NONE', #22217, #30230, #6885 ) ;
#14300=EDGE_CURVE ( 'NONE', #536, #8949, #11520, .T. ) ;
#14316=ADVANCED_FACE ( 'NONE', ( #10288 ), #20667, .T. ) ;
#14339=DIRECTION ( 'NONE',  ( -1.000000000000000000, 0.000000000000000000, 0.000000000000000000 ) ) ;
#14349=CIRCLE ( 'NONE', #4548, 100.0000000000000000 ) ;
#14519=ADVANCED_FACE ( 'NONE', ( #6143 ), #28993, .T. ) ;
#14561=VERTEX_POINT ( 'NONE', #21488 ) ;
#14564=CIRCLE ( 'NONE', #4221, 2.149999999999985256 ) ;
#14615=ORIENTED_EDGE ( 'NONE', *, *, #7494, .T. ) ;
#14631=CYLINDRICAL_SURFACE ( 'NONE', #26018, 13.50000000000001066 ) ;
#14656=EDGE_LOOP ( 'NONE', ( #15201, #11633, #19223, #9201 ) ) ;
#14724=LINE ( 'NONE', #22568, #30859 ) ;
#14768=ADVANCED_FACE ( 'NONE', ( #8966 ), #673, .T. ) ;
#14801=AXIS2_PLACEMENT_3D ( 'NONE', #26685, #14075, #32303 ) ;
#14873=CIRCLE ( 'NONE', #9977, 2.149999999999979483 ) ;
#14919=EDGE_CURVE ( 'NONE', #6813, #3136, #7200, .T. ) ;
#14938=DIRECTION ( 'NONE',  ( -1.000000000000000000, -0.000000000000000000, -0.000000000000000000 ) ) ;
#14968=ADVANCED_FACE ( 'NONE', ( #9299 ), #9636, .F. ) ;
#14983=ORIENTED_EDGE ( 'NONE', *, *, #4964, .F. ) ;
#14985=EDGE_CURVE ( 'NONE', #33036, #30420, #24065, .T. ) ;
#15008=CARTESIAN_POINT ( 'NONE',  ( 117.5000000000000000, 258.9084171661918958, -28.95509836041982510 ) ) ;
#15030=DIRECTION ( 'NONE',  ( 0.000000000000000000, 0.000000000000000000, 1.000000000000000000 ) ) ;
#15039=CARTESIAN_POINT ( 'NONE',  ( 117.5000000000000000, 207.9999999999998010, -93.94869280115065635 ) ) ;
#15058=AXIS2_PLACEMENT_3D ( 'NONE', #31339, #33396, #7 ) ;
#15066=CARTESIAN_POINT ( 'NONE',  ( 115.4999999999999858, 102.0000000000001990, 89.64869280115065919 ) ) ;
#15067=EDGE_LOOP ( 'NONE', ( #13939, #6984 ) ) ;
#15086=CARTESIAN_POINT ( 'NONE',  ( 115.4999999999999858, 207.9999999999998010, -93.94869280115064214 ) ) ;
#15188=CYLINDRICAL_SURFACE ( 'NONE', #19515, 15.50000000000001066 ) ;
#15200=DIRECTION ( 'NONE',  ( 0.000000000000000000, 0.7071067811865442421, -0.7071067811865506814 ) ) ;
#15201=ORIENTED_EDGE ( 'NONE', *, *, #17707, .F. ) ;
#15231=AXIS2_PLACEMENT_3D ( 'NONE', #27915, #12247, #31450 ) ;
#15317=EDGE_LOOP ( 'NONE', ( #5102, #17532, #12838, #4566 ) ) ;
#15323=ORIENTED_EDGE ( 'NONE', *, *, #26257, .F. ) ;
#15332=VECTOR ( 'NONE', #20792, 1000.000000000000000 ) ;
#15353=EDGE_CURVE ( 'NONE', #2045, #10532, #4499, .T. ) ;
#15401=ORIENTED_EDGE ( 'NONE', *, *, #23707, .T. ) ;
#15410=CARTESIAN_POINT ( 'NONE',  ( 107.5000000000000000, 155.0000000000000000, 100.0000000000000000 ) ) ;
#15421=FACE_OUTER_BOUND ( 'NONE', #1073, .T. ) ;
#15423=CARTESIAN_POINT ( 'NONE',  ( 77.50000000000000000, 155.0000000000000000, -6.938893903907228378E-15 ) ) ;
#15466=CIRCLE ( 'NONE', #26883, 27.99999999999999645 ) ;
#15540=ORIENTED_EDGE ( 'NONE', *, *, #11204, .T. ) ;
#15548=DIRECTION ( 'NONE',  ( 1.000000000000000000, 0.000000000000000000, 0.000000000000000000 ) ) ;
#15569=EDGE_CURVE ( 'NONE', #21649, #16763, #2340, .T. ) ;
#15577=EDGE_CURVE ( 'NONE', #31166, #27139, #33343, .T. ) ;
#15587=VECTOR ( 'NONE', #5303, 1000.000000000000114 ) ;
#15609=FACE_OUTER_BOUND ( 'NONE', #31384, .T. ) ;
#15624=CIRCLE ( 'NONE', #31930, 15.50000000000001066 ) ;
#15657=VERTEX_POINT ( 'NONE', #26130 ) ;
#15695=ORIENTED_EDGE ( 'NONE', *, *, #12672, .T. ) ;
#15708=DIRECTION ( 'NONE',  ( 1.000000000000000000, 0.000000000000000000, 0.000000000000000000 ) ) ;
#15710=CIRCLE ( 'NONE', #13022, 30.00000000000000000 ) ;
#15736=DIRECTION ( 'NONE',  ( 0.000000000000000000, 0.000000000000000000, -1.000000000000000000 ) ) ;
#15748=ORIENTED_EDGE ( 'NONE', *, *, #3082, .T. ) ;
#15792=CARTESIAN_POINT ( 'NONE',  ( 115.4999999999999858, 183.9550983604194698, 103.9084171661920095 ) ) ;
#15797=DIRECTION ( 'NONE',  ( 0.000000000000000000, 0.000000000000000000, -1.000000000000000000 ) ) ;
#15805=FACE_BOUND ( 'NONE', #1450, .T. ) ;
#15818=ORIENTED_EDGE ( 'NONE', *, *, #10995, .F. ) ;
#15821=ORIENTED_EDGE ( 'NONE', *, *, #8901, .T. ) ;
#15833=( NAMED_UNIT ( * ) SI_UNIT ( $, .STERADIAN. ) SOLID_ANGLE_UNIT ( ) );
#15881=DIRECTION ( 'NONE',  ( 1.000000000000000000, 0.000000000000000000, 0.000000000000000000 ) ) ;
#15886=DIRECTION ( 'NONE',  ( 0.000000000000000000, 0.7071067811865330288, -0.7071067811865621167 ) ) ;
#15891=DIRECTION ( 'NONE',  ( 0.000000000000000000, 0.000000000000000000, -1.000000000000000000 ) ) ;
#15906=EDGE_CURVE ( 'NONE', #16399, #536, #16226, .T. ) ;
#15916=VECTOR ( 'NONE', #3280, 1000.000000000000000 ) ;
#15931=EDGE_LOOP ( 'NONE', ( #27512, #438, #30716, #20660 ) ) ;
#15945=CARTESIAN_POINT ( 'NONE',  ( 117.5000000000000000, 155.0000000000000000, -6.938893903907228378E-15 ) ) ;
#15949=CIRCLE ( 'NONE', #6139, 2.149999999999985256 ) ;
#15974=AXIS2_PLACEMENT_3D ( 'NONE', #26102, #18096, #28821 ) ;
#15989=EDGE_LOOP ( 'NONE', ( #32565, #19881, #14615, #22944 ) ) ;
#15992=DIRECTION ( 'NONE',  ( 0.9396926207859072067, 0.000000000000000000, -0.3420201433256717105 ) ) ;
#16010=LINE ( 'NONE', #3227, #8390 ) ;
#16038=ORIENTED_EDGE ( 'NONE', *, *, #14985, .T. ) ;
#16040=CARTESIAN_POINT ( 'NONE',  ( 115.4999999999999858, 155.0000000000000000, -6.938893903907228378E-15 ) ) ;
#16064=ORIENTED_EDGE ( 'NONE', *, *, #23687, .T. ) ;
#16114=( LENGTH_UNIT ( ) NAMED_UNIT ( * ) SI_UNIT ( .MILLI., .METRE. ) );
#16121=CARTESIAN_POINT ( 'NONE',  ( 77.50000000000000000, 155.0000000000000000, -6.938893903907228378E-15 ) ) ;
#16226=LINE ( 'NONE', #32070, #15916 ) ;
#16264=AXIS2_PLACEMENT_3D ( 'NONE', #17441, #11827, #24606 ) ;
#16319=CYLINDRICAL_SURFACE ( 'NONE', #6215, 2.150000000000004352 ) ;
#16325=( LENGTH_UNIT ( ) NAMED_UNIT ( * ) SI_UNIT ( .MILLI., .METRE. ) );
#16346=ORIENTED_EDGE ( 'NONE', *, *, #23687, .F. ) ;
#16382=ORIENTED_EDGE ( 'NONE', *, *, #4719, .T. ) ;
#16399=VERTEX_POINT ( 'NONE', #20473 ) ;
#16438=ORIENTED_EDGE ( 'NONE', *, *, #7107, .F. ) ;
#16446=AXIS2_PLACEMENT_3D ( 'NONE', #6892, #20350, #9963 ) ;
#16492=CIRCLE ( 'NONE', #13773, 2.149999999999996803 ) ;
#16530=ADVANCED_BREP_SHAPE_REPRESENTATION ( '', ( #1232, #2404 ), #33431 ) ;
#16556=CARTESIAN_POINT ( 'NONE',  ( 77.50000000000000000, 155.0000000000000000, -7.500000000000022204 ) ) ;
#16611=ORIENTED_EDGE ( 'NONE', *, *, #33299, .T. ) ;
#16618=( NAMED_UNIT ( * ) SI_UNIT ( $, .STERADIAN. ) SOLID_ANGLE_UNIT ( ) );
#16649=AXIS2_PLACEMENT_3D ( 'NONE', #3984, #14205, #11488 ) ;
#16651=CARTESIAN_POINT ( 'NONE',  ( 115.4999999999999858, 155.0000000000000000, -6.938893903907228378E-15 ) ) ;
#16763=VERTEX_POINT ( 'NONE', #10757 ) ;
#16792=AXIS2_PLACEMENT_3D ( 'NONE', #6026, #32264, #5862 ) ;
#16795=EDGE_CURVE ( 'NONE', #8949, #536, #9930, .T. ) ;
#16798=CYLINDRICAL_SURFACE ( 'NONE', #25485, 2.149999999999999023 ) ;
#16824=FACE_BOUND ( 'NONE', #27168, .T. ) ;
#16832=CARTESIAN_POINT ( 'NONE',  ( 77.50000000000000000, 155.0000000000000000, 7.500000000000007994 ) ) ;
#16919=DIRECTION ( 'NONE',  ( 1.000000000000000000, 0.000000000000000000, 0.000000000000000000 ) ) ;
#17022=ORIENTED_EDGE ( 'NONE', *, *, #21749, .T. ) ;
#17035=EDGE_LOOP ( 'NONE', ( #18287, #20316, #28351, #24232 ) ) ;
#17038=LINE ( 'NONE', #7160, #21038 ) ;
#17137=DIRECTION ( 'NONE',  ( -1.000000000000000000, -0.000000000000000000, -0.000000000000000000 ) ) ;
#17162=DIRECTION ( 'NONE',  ( 0.000000000000000000, 0.000000000000000000, -1.000000000000000000 ) ) ;
#17244=DIRECTION ( 'NONE',  ( 0.000000000000000000, 0.000000000000000000, -1.000000000000000000 ) ) ;
#17251=VECTOR ( 'NONE', #20022, 1000.000000000000000 ) ;
#17252=ORIENTED_EDGE ( 'NONE', *, *, #13514, .F. ) ;
#17265=CARTESIAN_POINT ( 'NONE',  ( 77.50000000000000000, 155.0000000000000000, 13.50000000000000355 ) ) ;
#17271=AXIS2_PLACEMENT_3D ( 'NONE', #24602, #30392, #11658 ) ;
#17279=EDGE_LOOP ( 'NONE', ( #9965, #32961 ) ) ;
#17295=ORIENTED_EDGE ( 'NONE', *, *, #7924, .T. ) ;
#17310=DIRECTION ( 'NONE',  ( 1.000000000000000000, -0.000000000000000000, -0.000000000000000000 ) ) ;
#17330=ORIENTED_EDGE ( 'NONE', *, *, #4490, .T. ) ;
#17421=EDGE_LOOP ( 'NONE', ( #6567, #27624, #7831, #16438 ) ) ;
#17424=EDGE_CURVE ( 'NONE', #13306, #33027, #20278, .T. ) ;
#17441=CARTESIAN_POINT ( 'NONE',  ( 121.3406204335659879, 155.0000000000000000, -6.938893903907228378E-15 ) ) ;
#17451=DIRECTION ( 'NONE',  ( -1.000000000000000000, 0.000000000000000000, -0.000000000000000000 ) ) ;
#17491=AXIS2_PLACEMENT_3D ( 'NONE', #27995, #27652, #20331 ) ;
#17503=EDGE_CURVE ( 'NONE', #16763, #21649, #9958, .T. ) ;
#17511=CARTESIAN_POINT ( 'NONE',  ( 115.4999999999999858, 246.7986928011511907, 52.99999999999882760 ) ) ;
#17532=ORIENTED_EDGE ( 'NONE', *, *, #11366, .T. ) ;
#17538=EDGE_LOOP ( 'NONE', ( #9240, #33261, #8619, #27469 ) ) ;
#17581=VECTOR ( 'NONE', #5347, 1000.000000000000000 ) ;
#17584=AXIS2_PLACEMENT_3D ( 'NONE', #26348, #3010, #8292 ) ;
#17586=ORIENTED_EDGE ( 'NONE', *, *, #12723, .F. ) ;
#17628=AXIS2_PLACEMENT_3D ( 'NONE', #28760, #26195, #7477 ) ;
#17667=VERTEX_POINT ( 'NONE', #22738 ) ;
#17694=FACE_BOUND ( 'NONE', #27295, .T. ) ;
#17707=EDGE_CURVE ( 'NONE', #6813, #31166, #20517, .T. ) ;
#17710=ORIENTED_EDGE ( 'NONE', *, *, #21435, .F. ) ;
#17831=CIRCLE ( 'NONE', #24371, 2.149999999999999023 ) ;
#17886=PRODUCT ( 'air chamber shell rear', 'air chamber shell rear', '', ( #670 ) ) ;
#17916=EDGE_CURVE ( 'NONE', #21928, #10681, #7406, .T. ) ;
#17929=CYLINDRICAL_SURFACE ( 'NONE', #30830, 2.149999999999999023 ) ;
#17934=ORIENTED_EDGE ( 'NONE', *, *, #32890, .F. ) ;
#17951=EDGE_CURVE ( 'NONE', #30420, #33036, #20307, .T. ) ;
#17971=ORIENTED_EDGE ( 'NONE', *, *, #21749, .F. ) ;
#17979=CARTESIAN_POINT ( 'NONE',  ( 115.4999999999999858, 207.9999999999998010, -93.94869280115065635 ) ) ;
#18015=CARTESIAN_POINT ( 'NONE',  ( 121.3406204335659879, 155.0000000000000000, -7.500000000000022204 ) ) ;
#18017=CIRCLE ( 'NONE', #19638, 100.0000000000000000 ) ;
#18036=EDGE_CURVE ( 'NONE', #28279, #20901, #27347, .T. ) ;
#18041=AXIS2_PLACEMENT_3D ( 'NONE', #23888, #24049, #21827 ) ;
#18061=DIRECTION ( 'NONE',  ( 0.000000000000000000, -0.7071067811865346942, 0.7071067811865604513 ) ) ;
#18074=CARTESIAN_POINT ( 'NONE',  ( 115.4999999999999858, 244.6486928011512134, 52.99999999999884892 ) ) ;
#18096=DIRECTION ( 'NONE',  ( 1.000000000000000000, 0.000000000000000000, 0.000000000000000000 ) ) ;
#18098=AXIS2_PLACEMENT_3D ( 'NONE', #7557, #31061, #28332 ) ;
#18123=FACE_OUTER_BOUND ( 'NONE', #4125, .T. ) ;
#18136=ADVANCED_FACE ( 'NONE', ( #10965 ), #24410, .F. ) ;
#18251=CARTESIAN_POINT ( 'NONE',  ( 77.50000000000000000, 155.0000000000000000, -70.00000000000000000 ) ) ;
#18277=CARTESIAN_POINT ( 'NONE',  ( 115.4999999999999858, 155.0000000000000000, 112.0000000000000426 ) ) ;
#18287=ORIENTED_EDGE ( 'NONE', *, *, #23034, .F. ) ;
#18288=CARTESIAN_POINT ( 'NONE',  ( 115.4999999999999858, 65.35130719884917028, -52.99999999999947420 ) ) ;
#18309=ORIENTED_EDGE ( 'NONE', *, *, #15569, .F. ) ;
#18357=DIRECTION ( 'NONE',  ( -1.000000000000000000, 0.000000000000000000, 0.000000000000000000 ) ) ;
#18391=AXIS2_PLACEMENT_3D ( 'NONE', #21351, #31747, #1414 ) ;
#18447=LINE ( 'NONE', #18277, #29010 ) ;
#18469=ADVANCED_FACE ( 'NONE', ( #32283, #9112 ), #22062, .T. ) ;
#18470=CIRCLE ( 'NONE', #29895, 13.49999999999996980 ) ;
#18479=DIRECTION ( 'NONE',  ( 1.000000000000000000, 0.000000000000000000, 0.000000000000000000 ) ) ;
#18488=AXIS2_PLACEMENT_3D ( 'NONE', #30480, #7142, #31287 ) ;
#18515=EDGE_LOOP ( 'NONE', ( #32044, #20696 ) ) ;
#18524=DIRECTION ( 'NONE',  ( 0.000000000000000000, -1.000000000000000000, 3.227392513445223895E-15 ) ) ;
#18565=FILL_AREA_STYLE ('',( #26717 ) ) ;
#18566=CYLINDRICAL_SURFACE ( 'NONE', #7588, 2.149999999999979483 ) ;
#18592=DIRECTION ( 'NONE',  ( -1.000000000000000000, 0.000000000000000000, 0.000000000000000000 ) ) ;
#18599=VERTEX_POINT ( 'NONE', #15066 ) ;
#18604=ORIENTED_EDGE ( 'NONE', *, *, #4398, .F. ) ;
#18673=ORIENTED_EDGE ( 'NONE', *, *, #10323, .F. ) ;
#18693=CARTESIAN_POINT ( 'NONE',  ( 117.5000000000000000, 207.9999999999998010, -91.79869280115066488 ) ) ;
#18807=CARTESIAN_POINT ( 'NONE',  ( 77.50000000000000000, 155.0000000000000000, -6.938893903907228378E-15 ) ) ;
#18824=EDGE_LOOP ( 'NONE', ( #13434, #283, #17330, #27582 ) ) ;
#18851=CIRCLE ( 'NONE', #25375, 2.150000000000004352 ) ;
#18870=VERTEX_POINT ( 'NONE', #15410 ) ;
#18881=CARTESIAN_POINT ( 'NONE',  ( 115.4999999999999858, 127.5651812191323557, -102.3881375866411645 ) ) ;
#18906=CIRCLE ( 'NONE', #28714, 2.149999999999979483 ) ;
#18946=AXIS2_PLACEMENT_3D ( 'NONE', #28699, #18479, #29368 ) ;
#18954=CARTESIAN_POINT ( 'NONE',  ( 117.5000000000000000, 52.61186241335891367, 27.43481878086798176 ) ) ;
#18971=EDGE_CURVE ( 'NONE', #7638, #18870, #14349, .T. ) ;
#18991=DIRECTION ( 'NONE',  ( -1.000000000000000000, -0.000000000000000000, -0.000000000000000000 ) ) ;
#19006=ORIENTED_EDGE ( 'NONE', *, *, #8945, .F. ) ;
#19049=DIRECTION ( 'NONE',  ( -1.000000000000000000, -0.000000000000000000, 0.000000000000000000 ) ) ;
#19057=DIRECTION ( 'NONE',  ( 1.000000000000000000, 0.000000000000000000, 0.000000000000000000 ) ) ;
#19124=CIRCLE ( 'NONE', #7166, 2.149999999999974598 ) ;
#19126=DIRECTION ( 'NONE',  ( -1.000000000000000000, 0.000000000000000000, -0.000000000000000000 ) ) ;
#19128=ORIENTED_EDGE ( 'NONE', *, *, #29372, .T. ) ;
#19173=EDGE_CURVE ( 'NONE', #13672, #22445, #27936, .T. ) ;
#19174=ORIENTED_EDGE ( 'NONE', *, *, #3252, .T. ) ;
#19217=DIRECTION ( 'NONE',  ( 0.000000000000000000, 0.7071067811865506814, 0.7071067811865442421 ) ) ;
#19223=ORIENTED_EDGE ( 'NONE', *, *, #7683, .T. ) ;
#19225=AXIS2_PLACEMENT_3D ( 'NONE', #31473, #29076, #625 ) ;
#19226=LINE ( 'NONE', #29622, #23220 ) ;
#19257=ORIENTED_EDGE ( 'NONE', *, *, #4252, .F. ) ;
#19274=CARTESIAN_POINT ( 'NONE',  ( 115.4999999999999858, 182.4348187808683690, 102.3881375866409513 ) ) ;
#19311=DIRECTION ( 'NONE',  ( -1.000000000000000000, -0.000000000000000000, -0.000000000000000000 ) ) ;
#19362=EDGE_CURVE ( 'NONE', #11329, #6902, #1817, .T. ) ;
#19371=CARTESIAN_POINT ( 'NONE',  ( 77.50000000000000000, 155.0000000000000000, -6.938893903907228378E-15 ) ) ;
#19405=CIRCLE ( 'NONE', #29206, 2.149999999999994138 ) ;
#19451=CARTESIAN_POINT ( 'NONE',  ( 117.5000000000000000, 102.0000000000001990, 89.64869280115064498 ) ) ;
#19460=STYLED_ITEM ( 'NONE', ( #28907 ), #1232 ) ;
#19482=CIRCLE ( 'NONE', #27622, 30.00000000000000000 ) ;
#19487=LINE ( 'NONE', #9091, #1973 ) ;
#19510=DIRECTION ( 'NONE',  ( 0.000000000000000000, 0.000000000000000000, -1.000000000000000000 ) ) ;
#19511=ORIENTED_EDGE ( 'NONE', *, *, #23883, .T. ) ;
#19515=AXIS2_PLACEMENT_3D ( 'NONE', #9741, #27788, #25404 ) ;
#19529=EDGE_CURVE ( 'NONE', #2045, #21331, #11628, .T. ) ;
#19548=EDGE_LOOP ( 'NONE', ( #5136, #5965 ) ) ;
#19553=ADVANCED_FACE ( 'NONE', ( #2601 ), #4008, .T. ) ;
#19574=DIRECTION ( 'NONE',  ( 0.000000000000000000, 0.000000000000000000, -1.000000000000000000 ) ) ;
#19592=SHAPE_REPRESENTATION ( 'air chamber shell rear', ( #2404 ), #33431 ) ;
#19604=EDGE_LOOP ( 'NONE', ( #7918, #7451, #19174, #19128 ) ) ;
#19635=CIRCLE ( 'NONE', #24521, 7.500000000000015099 ) ;
#19638=AXIS2_PLACEMENT_3D ( 'NONE', #27392, #29958, #20235 ) ;
#19691=DIRECTION ( 'NONE',  ( -1.000000000000000000, -0.000000000000000000, -0.000000000000000000 ) ) ;
#19709=AXIS2_PLACEMENT_3D ( 'NONE', #30084, #19691, #32636 ) ;
#19717=FACE_BOUND ( 'NONE', #17279, .T. ) ;
#19768=CIRCLE ( 'NONE', #17584, 7.500000000000015099 ) ;
#19881=ORIENTED_EDGE ( 'NONE', *, *, #17951, .F. ) ;
#19883=FACE_BOUND ( 'NONE', #25969, .T. ) ;
#19918=VERTEX_POINT ( 'NONE', #4604 ) ;
#20022=DIRECTION ( 'NONE',  ( -1.000000000000000000, -0.000000000000000000, -0.000000000000000000 ) ) ;
#20063=ORIENTED_EDGE ( 'NONE', *, *, #1371, .F. ) ;
#20096=ORIENTED_EDGE ( 'NONE', *, *, #4719, .F. ) ;
#20110=DIRECTION ( 'NONE',  ( -1.000000000000000000, 0.000000000000000000, 0.000000000000000000 ) ) ;
#20184=EDGE_LOOP ( 'NONE', ( #2733, #12165, #30964, #14983 ) ) ;
#20229=FILL_AREA_STYLE ('',( #26024 ) ) ;
#20235=DIRECTION ( 'NONE',  ( 0.000000000000000000, 0.000000000000000000, -1.000000000000000000 ) ) ;
#20245=CARTESIAN_POINT ( 'NONE',  ( 115.4999999999999858, 258.9084171661918958, -28.95509836041981089 ) ) ;
#20254=AXIS2_PLACEMENT_3D ( 'NONE', #961, #8793, #24470 ) ;
#20255=ORIENTED_EDGE ( 'NONE', *, *, #16795, .F. ) ;
#20272=ORIENTED_EDGE ( 'NONE', *, *, #22842, .F. ) ;
#20278=CIRCLE ( 'NONE', #28988, 2.149999999999974598 ) ;
#20295=CARTESIAN_POINT ( 'NONE',  ( 107.5000000000000000, 155.0000000000000000, -6.938893903907228378E-15 ) ) ;
#20307=CIRCLE ( 'NONE', #27911, 70.00000000000000000 ) ;
#20316=ORIENTED_EDGE ( 'NONE', *, *, #21435, .T. ) ;
#20331=DIRECTION ( 'NONE',  ( 0.000000000000000000, 0.7071067811865475727, 0.7071067811865475727 ) ) ;
#20350=DIRECTION ( 'NONE',  ( 1.000000000000000000, 0.000000000000000000, 0.000000000000000000 ) ) ;
#20414=EDGE_CURVE ( 'NONE', #31059, #5646, #2953, .T. ) ;
#20462=CARTESIAN_POINT ( 'NONE',  ( 67.50000000000000000, 155.0000000000000000, -6.938893903907228378E-15 ) ) ;
#20473=CARTESIAN_POINT ( 'NONE',  ( 117.5000000000000000, 248.9486928011511679, 52.99999999999880629 ) ) ;
#20517=LINE ( 'NONE', #25802, #12642 ) ;
#20558=DIRECTION ( 'NONE',  ( -1.000000000000000000, 0.000000000000000000, 0.000000000000000000 ) ) ;
#20561=MECHANICAL_DESIGN_GEOMETRIC_PRESENTATION_REPRESENTATION('',(#19460),#22751);
#20583=DIRECTION ( 'NONE',  ( 0.000000000000000000, -1.000000000000000000, 9.682177540335733218E-15 ) ) ;
#20587=ADVANCED_FACE ( 'NONE', ( #31823 ), #13766, .F. ) ;
#20597=DIRECTION ( 'NONE',  ( 0.000000000000000000, -0.7071067811865506814, -0.7071067811865442421 ) ) ;
#20604=ADVANCED_FACE ( 'NONE', ( #5926 ), #16319, .F. ) ;
#20621=ORIENTED_EDGE ( 'NONE', *, *, #3894, .T. ) ;
#20645=EDGE_LOOP ( 'NONE', ( #5016, #13108, #17022, #4762 ) ) ;
#20649=ADVANCED_FACE ( 'NONE', ( #27727 ), #9497, .F. ) ;
#20660=ORIENTED_EDGE ( 'NONE', *, *, #434, .F. ) ;
#20667=CYLINDRICAL_SURFACE ( 'NONE', #18098, 99.99999999999997158 ) ;
#20694=ORIENTED_EDGE ( 'NONE', *, *, #18036, .T. ) ;
#20696=ORIENTED_EDGE ( 'NONE', *, *, #11894, .F. ) ;
#20701=DIRECTION ( 'NONE',  ( -1.000000000000000000, 0.000000000000000000, 0.000000000000000000 ) ) ;
#20706=CARTESIAN_POINT ( 'NONE',  ( 67.50000000000000000, 155.0000000000000000, -6.938893903907228378E-15 ) ) ;
#20724=EDGE_CURVE ( 'NONE', #6902, #11329, #776, .T. ) ;
#20736=CIRCLE ( 'NONE', #7145, 2.149999999999999023 ) ;
#20753=FACE_BOUND ( 'NONE', #28856, .T. ) ;
#20792=DIRECTION ( 'NONE',  ( -1.000000000000000000, 0.000000000000000000, -0.000000000000000000 ) ) ;
#20806=DIRECTION ( 'NONE',  ( 1.000000000000000000, 0.000000000000000000, 0.000000000000000000 ) ) ;
#20815=AXIS2_PLACEMENT_3D ( 'NONE', #16040, #13484, #21815 ) ;
#20823=CARTESIAN_POINT ( 'NONE',  ( 115.4999999999999858, 246.7986928011511907, 52.99999999999882760 ) ) ;
#20838=EDGE_CURVE ( 'NONE', #18599, #1916, #26812, .T. ) ;
#20841=ORIENTED_EDGE ( 'NONE', *, *, #3709, .F. ) ;
#20856=ORIENTED_EDGE ( 'NONE', *, *, #25399, .T. ) ;
#20889=CYLINDRICAL_SURFACE ( 'NONE', #18488, 97.99999999999997158 ) ;
#20901=VERTEX_POINT ( 'NONE', #28241 ) ;
#20917=AXIS2_PLACEMENT_3D ( 'NONE', #18881, #29274, #19217 ) ;
#20938=CARTESIAN_POINT ( 'NONE',  ( 115.4999999999999858, 182.4348187808683690, 102.3881375866409513 ) ) ;
#20970=LINE ( 'NONE', #2914, #3230 ) ;
#20988=VERTEX_POINT ( 'NONE', #25853 ) ;
#21006=ORIENTED_EDGE ( 'NONE', *, *, #14919, .F. ) ;
#21038=VECTOR ( 'NONE', #7340, 1000.000000000000000 ) ;
#21072=FACE_OUTER_BOUND ( 'NONE', #32451, .T. ) ;
#21088=AXIS2_PLACEMENT_3D ( 'NONE', #27717, #20558, #6935 ) ;
#21114=CARTESIAN_POINT ( 'NONE',  ( 115.4999999999999858, 257.3881375866408803, -27.43481878086871717 ) ) ;
#21126=CARTESIAN_POINT ( 'NONE',  ( 117.5000000000000000, 155.0000000000000000, -100.0000000000000000 ) ) ;
#21230=CARTESIAN_POINT ( 'NONE',  ( 117.5000000000000000, 246.7986928011511907, 52.99999999999882760 ) ) ;
#21234=EDGE_CURVE ( 'NONE', #19918, #16399, #15949, .T. ) ;
#21235=EDGE_CURVE ( 'NONE', #10430, #7925, #19768, .T. ) ;
#21277=( NAMED_UNIT ( * ) PLANE_ANGLE_UNIT ( ) SI_UNIT ( $, .RADIAN. ) );
#21306=DIRECTION ( 'NONE',  ( 1.000000000000000000, 0.000000000000000000, 0.000000000000000000 ) ) ;
#21331=VERTEX_POINT ( 'NONE', #9415 ) ;
#21343=ORIENTED_EDGE ( 'NONE', *, *, #11189, .T. ) ;
#21351=CARTESIAN_POINT ( 'NONE',  ( 117.5000000000000000, 155.0000000000000000, -6.938893903907228378E-15 ) ) ;
#21387=ORIENTED_EDGE ( 'NONE', *, *, #21669, .T. ) ;
#21435=EDGE_CURVE ( 'NONE', #30624, #30017, #11073, .T. ) ;
#21469=ORIENTED_EDGE ( 'NONE', *, *, #23908, .T. ) ;
#21488=CARTESIAN_POINT ( 'NONE',  ( 77.50000000000000000, 155.0000000000000000, 15.50000000000000355 ) ) ;
#21554=EDGE_CURVE ( 'NONE', #17667, #31655, #3599, .T. ) ;
#21557=CARTESIAN_POINT ( 'NONE',  ( 121.3406204335659879, 155.0000000000000000, 7.500000000000007994 ) ) ;
#21591=ORIENTED_EDGE ( 'NONE', *, *, #29173, .T. ) ;
#21614=AXIS2_PLACEMENT_3D ( 'NONE', #24940, #8926, #6365 ) ;
#21631=ORIENTED_EDGE ( 'NONE', *, *, #7954, .T. ) ;
#21649=VERTEX_POINT ( 'NONE', #27490 ) ;
#21669=EDGE_CURVE ( 'NONE', #6902, #31655, #950, .T. ) ;
#21735=DIRECTION ( 'NONE',  ( 1.000000000000000000, 0.000000000000000000, 0.000000000000000000 ) ) ;
#21749=EDGE_CURVE ( 'NONE', #31748, #13306, #19487, .T. ) ;
#21767=AXIS2_PLACEMENT_3D ( 'NONE', #8181, #25727, #18061 ) ;
#21774=DIRECTION ( 'NONE',  ( 1.000000000000000000, 0.000000000000000000, 0.000000000000000000 ) ) ;
#21789=EDGE_CURVE ( 'NONE', #27139, #31166, #6319, .T. ) ;
#21792=DIRECTION ( 'NONE',  ( 1.000000000000000000, 0.000000000000000000, 0.000000000000000000 ) ) ;
#21815=DIRECTION ( 'NONE',  ( 0.000000000000000000, 0.000000000000000000, -1.000000000000000000 ) ) ;
#21827=DIRECTION ( 'NONE',  ( 0.000000000000000000, 0.000000000000000000, -1.000000000000000000 ) ) ;
#21870=FACE_OUTER_BOUND ( 'NONE', #14656, .T. ) ;
#21896=VECTOR ( 'NONE', #12335, 1000.000000000000000 ) ;
#21928=VERTEX_POINT ( 'NONE', #7571 ) ;
#21945=CARTESIAN_POINT ( 'NONE',  ( 115.4999999999999858, 61.05130719884918733, -52.99999999999945999 ) ) ;
#22032=CARTESIAN_POINT ( 'NONE',  ( 77.50000000000000000, 155.0000000000000000, -6.938893903907228378E-15 ) ) ;
#22062=PLANE ( 'NONE',  #3983 ) ;
#22106=CARTESIAN_POINT ( 'NONE',  ( 79.50000000000000000, 155.0000000000000000, -6.938893903907228378E-15 ) ) ;
#22124=DIRECTION ( 'NONE',  ( -1.000000000000000000, -0.000000000000000000, -0.000000000000000000 ) ) ;
#22132=ORIENTED_EDGE ( 'NONE', *, *, #26000, .T. ) ;
#22167=CARTESIAN_POINT ( 'NONE',  ( 117.5000000000000000, 155.0000000000000000, 112.0000000000000426 ) ) ;
#22193=FACE_OUTER_BOUND ( 'NONE', #12895, .T. ) ;
#22217=CARTESIAN_POINT ( 'NONE',  ( 115.4999999999999858, 63.20130719884917170, -52.99999999999946709 ) ) ;
#22219=ORIENTED_EDGE ( 'NONE', *, *, #3737, .T. ) ;
#22234=EDGE_LOOP ( 'NONE', ( #23164, #27008, #3166, #17252 ) ) ;
#22267=ORIENTED_EDGE ( 'NONE', *, *, #10985, .F. ) ;
#22367=DIRECTION ( 'NONE',  ( 0.000000000000000000, -0.7071067811865540120, -0.7071067811865411334 ) ) ;
#22400=CIRCLE ( 'NONE', #32736, 100.0000000000000000 ) ;
#22445=VERTEX_POINT ( 'NONE', #1230 ) ;
#22532=DIRECTION ( 'NONE',  ( -1.000000000000000000, 0.000000000000000000, 0.000000000000000000 ) ) ;
#22568=CARTESIAN_POINT ( 'NONE',  ( 77.50000000000000000, 155.0000000000000000, -13.50000000000001776 ) ) ;
#22575=CARTESIAN_POINT ( 'NONE',  ( 115.4999999999999858, 155.0000000000000000, -112.0000000000000426 ) ) ;
#22610=DIRECTION ( 'NONE',  ( 0.000000000000000000, 0.000000000000000000, -1.000000000000000000 ) ) ;
#22611=DIRECTION ( 'NONE',  ( -1.000000000000000000, 0.000000000000000000, 0.000000000000000000 ) ) ;
#22633=UNCERTAINTY_MEASURE_WITH_UNIT (LENGTH_MEASURE( 1.000000000000000082E-05 ), #506, 'distance_accuracy_value', 'NONE');
#22714=CARTESIAN_POINT ( 'NONE',  ( 117.5000000000000000, 52.61186241335891367, 27.43481878086798176 ) ) ;
#22738=CARTESIAN_POINT ( 'NONE',  ( 107.5000000000000000, 155.0000000000000000, -98.00000000000000000 ) ) ;
#22747=ORIENTED_EDGE ( 'NONE', *, *, #28534, .F. ) ;
#22751=( GEOMETRIC_REPRESENTATION_CONTEXT ( 3 ) GLOBAL_UNCERTAINTY_ASSIGNED_CONTEXT ( ( #29072 ) ) GLOBAL_UNIT_ASSIGNED_CONTEXT ( ( #16114, #5725, #16618 ) ) REPRESENTATION_CONTEXT ( 'NONE', 'WORKASPACE' ) );
#22781=EDGE_LOOP ( 'NONE', ( #32989, #19257 ) ) ;
#22809=FACE_OUTER_BOUND ( 'NONE', #32827, .T. ) ;
#22842=EDGE_CURVE ( 'NONE', #4349, #20988, #28142, .T. ) ;
#22857=ORIENTED_EDGE ( 'NONE', *, *, #14160, .T. ) ;
#22865=EDGE_CURVE ( 'NONE', #32282, #26009, #23742, .T. ) ;
#22866=EDGE_LOOP ( 'NONE', ( #5843, #18673 ) ) ;
#22898=ADVANCED_FACE ( 'NONE', ( #7874 ), #17929, .F. ) ;
#22910=CARTESIAN_POINT ( 'NONE',  ( 117.5000000000000000, 126.0449016395812691, -103.9084171661922369 ) ) ;
#22944=ORIENTED_EDGE ( 'NONE', *, *, #5023, .F. ) ;
#22962=CARTESIAN_POINT ( 'NONE',  ( 115.4999999999999858, 207.9999999999998010, -89.64869280115065919 ) ) ;
#22973=FACE_OUTER_BOUND ( 'NONE', #2077, .T. ) ;
#22987=EDGE_LOOP ( 'NONE', ( #18604, #19006, #31573, #32619 ) ) ;
#22990=ORIENTED_EDGE ( 'NONE', *, *, #19529, .F. ) ;
#23034=EDGE_CURVE ( 'NONE', #30624, #1916, #5473, .T. ) ;
#23041=ORIENTED_EDGE ( 'NONE', *, *, #28138, .T. ) ;
#23053=CARTESIAN_POINT ( 'NONE',  ( 115.4999999999999858, 182.4348187808683690, 102.3881375866409513 ) ) ;
#23123=ORIENTED_EDGE ( 'NONE', *, *, #17707, .T. ) ;
#23148=LINE ( 'NONE', #20245, #29289 ) ;
#23164=ORIENTED_EDGE ( 'NONE', *, *, #23707, .F. ) ;
#23184=LINE ( 'NONE', #18074, #15332 ) ;
#23220=VECTOR ( 'NONE', #9173, 1000.000000000000000 ) ;
#23355=CARTESIAN_POINT ( 'NONE',  ( 117.5000000000000000, 102.0000000000001990, 93.94869280115064214 ) ) ;
#23413=CARTESIAN_POINT ( 'NONE',  ( 77.50000000000000000, 155.0000000000000000, -6.938893903907228378E-15 ) ) ;
#23430=FACE_BOUND ( 'NONE', #14145, .T. ) ;
#23549=DIRECTION ( 'NONE',  ( 0.000000000000000000, -1.000000000000000000, 9.682177540335733218E-15 ) ) ;
#23560=CARTESIAN_POINT ( 'NONE',  ( 77.50000000000000000, 155.0000000000000000, -6.938893903907228378E-15 ) ) ;
#23563=DIRECTION ( 'NONE',  ( 1.000000000000000000, 0.000000000000000000, 0.000000000000000000 ) ) ;
#23613=AXIS2_PLACEMENT_3D ( 'NONE', #5279, #23675, #10411 ) ;
#23636=CARTESIAN_POINT ( 'NONE',  ( 117.5000000000000000, 255.8678580070898363, -25.91453920131760924 ) ) ;
#23675=DIRECTION ( 'NONE',  ( -1.000000000000000000, 0.000000000000000000, 0.000000000000000000 ) ) ;
#23682=DIRECTION ( 'NONE',  ( 0.000000000000000000, 0.000000000000000000, -1.000000000000000000 ) ) ;
#23687=EDGE_CURVE ( 'NONE', #10532, #33564, #19405, .T. ) ;
#23707=EDGE_CURVE ( 'NONE', #171, #14561, #9069, .T. ) ;
#23717=DIRECTION ( 'NONE',  ( 0.000000000000000000, -0.7071067811865506814, -0.7071067811865442421 ) ) ;
#23742=CIRCLE ( 'NONE', #349, 13.50000000000001066 ) ;
#23744=ORIENTED_EDGE ( 'NONE', *, *, #14300, .F. ) ;
#23759=CARTESIAN_POINT ( 'NONE',  ( 115.4999999999999858, 65.35130719884915607, -52.99999999999947420 ) ) ;
#23857=CARTESIAN_POINT ( 'NONE',  ( 115.4999999999999858, 246.7986928011511907, 52.99999999999882760 ) ) ;
#23883=EDGE_CURVE ( 'NONE', #12782, #25798, #27592, .T. ) ;
#23888=CARTESIAN_POINT ( 'NONE',  ( 115.4999999999999858, 102.0000000000001990, 91.79869280115065067 ) ) ;
#23905=CARTESIAN_POINT ( 'NONE',  ( 117.5000000000000000, 155.0000000000000000, -6.938893903907228378E-15 ) ) ;
#23908=EDGE_CURVE ( 'NONE', #6774, #15657, #8046, .T. ) ;
#23954=ORIENTED_EDGE ( 'NONE', *, *, #16795, .T. ) ;
#23974=CARTESIAN_POINT ( 'NONE',  ( 115.4999999999999858, 207.9999999999998010, -91.79869280115066488 ) ) ;
#23993=CARTESIAN_POINT ( 'NONE',  ( 117.5000000000000000, 207.9999999999998010, -91.79869280115066488 ) ) ;
#23999=EDGE_LOOP ( 'NONE', ( #8616, #22990 ) ) ;
#24049=DIRECTION ( 'NONE',  ( -1.000000000000000000, 0.000000000000000000, 0.000000000000000000 ) ) ;
#24065=CIRCLE ( 'NONE', #9377, 70.00000000000000000 ) ;
#24089=ADVANCED_FACE ( 'NONE', ( #15609 ), #13561, .T. ) ;
#24159=CARTESIAN_POINT ( 'NONE',  ( 72.99495483890930814, 155.0000000000000000, -15.50000000000001776 ) ) ;
#24232=ORIENTED_EDGE ( 'NONE', *, *, #20838, .T. ) ;
#24260=DIRECTION ( 'NONE',  ( 1.000000000000000000, 0.000000000000000000, 0.000000000000000000 ) ) ;
#24283=VECTOR ( 'NONE', #18592, 1000.000000000000000 ) ;
#24351=CIRCLE ( 'NONE', #3128, 13.49999999999996980 ) ;
#24371=AXIS2_PLACEMENT_3D ( 'NONE', #8140, #21735, #18524 ) ;
#24410=CYLINDRICAL_SURFACE ( 'NONE', #12671, 2.149999999999979483 ) ;
#24412=ORIENTED_EDGE ( 'NONE', *, *, #10985, .T. ) ;
#24436=DIRECTION ( 'NONE',  ( 0.000000000000000000, 0.000000000000000000, -1.000000000000000000 ) ) ;
#24470=DIRECTION ( 'NONE',  ( 0.000000000000000000, -1.000000000000000000, 3.227392513445223895E-15 ) ) ;
#24489=ORIENTED_EDGE ( 'NONE', *, *, #17951, .T. ) ;
#24502=ORIENTED_EDGE ( 'NONE', *, *, #31210, .F. ) ;
#24521=AXIS2_PLACEMENT_3D ( 'NONE', #20462, #26082, #13290 ) ;
#24566=VERTEX_POINT ( 'NONE', #22910 ) ;
#24575=CIRCLE ( 'NONE', #18041, 2.149999999999985256 ) ;
#24602=CARTESIAN_POINT ( 'NONE',  ( 115.4999999999999858, 63.20130719884917170, -52.99999999999946709 ) ) ;
#24606=DIRECTION ( 'NONE',  ( 0.000000000000000000, 0.000000000000000000, 1.000000000000000000 ) ) ;
#24643=CARTESIAN_POINT ( 'NONE',  ( 115.4999999999999858, 54.13214199290997186, 25.91453920131690936 ) ) ;
#24665=ORIENTED_EDGE ( 'NONE', *, *, #33511, .T. ) ;
#24667=FACE_OUTER_BOUND ( 'NONE', #2351, .T. ) ;
#24669=DIRECTION ( 'NONE',  ( 0.000000000000000000, -1.000000000000000000, 9.682177540335733218E-15 ) ) ;
#24681=ADVANCED_FACE ( 'NONE', ( #9619, #30417 ), #27095, .F. ) ;
#24691=CARTESIAN_POINT ( 'NONE',  ( 115.4999999999999858, 155.0000000000000000, -6.938893903907228378E-15 ) ) ;
#24695=CIRCLE ( 'NONE', #6178, 2.149999999999999023 ) ;
#24831=FACE_BOUND ( 'NONE', #22781, .T. ) ;
#24901=DIRECTION ( 'NONE',  ( 1.000000000000000000, 0.000000000000000000, 0.000000000000000000 ) ) ;
#24916=VECTOR ( 'NONE', #14339, 1000.000000000000000 ) ;
#24940=CARTESIAN_POINT ( 'NONE',  ( 107.5000000000000000, 155.0000000000000000, -6.938893903907228378E-15 ) ) ;
#24945=CARTESIAN_POINT ( 'NONE',  ( 107.5000000000000000, 155.0000000000000000, -70.00000000000000000 ) ) ;
#25005=FACE_BOUND ( 'NONE', #29606, .T. ) ;
#25024=CARTESIAN_POINT ( 'NONE',  ( 117.5000000000000000, 54.13214199290997897, 25.91453920131689515 ) ) ;
#25052=ORIENTED_EDGE ( 'NONE', *, *, #17424, .F. ) ;
#25061=TOROIDAL_SURFACE ( 'NONE', #31063, 69.99999999999998579, 30.00000000000000000 ) ;
#25094=DIRECTION ( 'NONE',  ( 1.000000000000000000, 0.000000000000000000, 0.000000000000000000 ) ) ;
#25105=CIRCLE ( 'NONE', #17491, 2.149999999999974598 ) ;
#25108=DIRECTION ( 'NONE',  ( 0.000000000000000000, 0.000000000000000000, -1.000000000000000000 ) ) ;
#25125=EDGE_CURVE ( 'NONE', #33036, #18870, #19482, .T. ) ;
#25163=FACE_BOUND ( 'NONE', #13810, .T. ) ;
#25164=DIRECTION ( 'NONE',  ( -1.000000000000000000, 0.000000000000000000, -0.000000000000000000 ) ) ;
#25203=ORIENTED_EDGE ( 'NONE', *, *, #7954, .F. ) ;
#25229=AXIS2_PLACEMENT_3D ( 'NONE', #13684, #13862, #26637 ) ;
#25335=CARTESIAN_POINT ( 'NONE',  ( 79.50000000000000000, 155.0000000000000000, -13.50000000000001776 ) ) ;
#25375=AXIS2_PLACEMENT_3D ( 'NONE', #6270, #21774, #23717 ) ;
#25399=EDGE_CURVE ( 'NONE', #5869, #13101, #26881, .T. ) ;
#25404=DIRECTION ( 'NONE',  ( 0.000000000000000000, 0.000000000000000000, 1.000000000000000000 ) ) ;
#25452=CIRCLE ( 'NONE', #29807, 112.0000000000000426 ) ;
#25461=ORIENTED_EDGE ( 'NONE', *, *, #15577, .F. ) ;
#25465=CIRCLE ( 'NONE', #18946, 2.149999999999994138 ) ;
#25485=AXIS2_PLACEMENT_3D ( 'NONE', #8634, #29588, #31639 ) ;
#25511=SURFACE_SIDE_STYLE ('',( #30630 ) ) ;
#25540=CIRCLE ( 'NONE', #4331, 2.149999999999996803 ) ;
#25560=CIRCLE ( 'NONE', #15231, 15.50000000000001066 ) ;
#25570=DIRECTION ( 'NONE',  ( 0.000000000000000000, -1.000000000000000000, 0.000000000000000000 ) ) ;
#25581=ORIENTED_EDGE ( 'NONE', *, *, #11366, .F. ) ;
#25617=DIRECTION ( 'NONE',  ( -1.000000000000000000, 0.000000000000000000, 0.000000000000000000 ) ) ;
#25679=AXIS2_PLACEMENT_3D ( 'NONE', #20823, #7890, #23549 ) ;
#25727=DIRECTION ( 'NONE',  ( -1.000000000000000000, 0.000000000000000000, -0.000000000000000000 ) ) ;
#25731=DIRECTION ( 'NONE',  ( 1.000000000000000000, 0.000000000000000000, 0.000000000000000000 ) ) ;
#25798=VERTEX_POINT ( 'NONE', #12051 ) ;
#25802=CARTESIAN_POINT ( 'NONE',  ( 115.4999999999999858, 61.05130719884917312, -52.99999999999945999 ) ) ;
#25824=ADVANCED_FACE ( 'NONE', ( #24831, #25163, #16824, #19717, #27381, #25005, #27219, #19883, #32830, #24667 ), #4047, .F. ) ;
#25853=CARTESIAN_POINT ( 'NONE',  ( 72.99495483890930814, 155.0000000000000000, 15.50000000000000355 ) ) ;
#25871=FACE_BOUND ( 'NONE', #14063, .T. ) ;
#25896=FACE_OUTER_BOUND ( 'NONE', #29187, .T. ) ;
#25969=EDGE_LOOP ( 'NONE', ( #4289, #13761 ) ) ;
#25988=DIRECTION ( 'NONE',  ( -1.000000000000000000, -0.000000000000000000, -0.000000000000000000 ) ) ;
#26000=EDGE_CURVE ( 'NONE', #7925, #12782, #27886, .T. ) ;
#26001=FACE_OUTER_BOUND ( 'NONE', #17421, .T. ) ;
#26009=VERTEX_POINT ( 'NONE', #25335 ) ;
#26018=AXIS2_PLACEMENT_3D ( 'NONE', #30137, #22124, #27744 ) ;
#26024=FILL_AREA_STYLE_COLOUR ( '', #30364 ) ;
#26057=EDGE_LOOP ( 'NONE', ( #13962, #26669, #5397, #31016 ) ) ;
#26082=DIRECTION ( 'NONE',  ( -1.000000000000000000, 0.000000000000000000, 0.000000000000000000 ) ) ;
#26085=DIRECTION ( 'NONE',  ( -1.000000000000000000, -0.000000000000000000, -0.000000000000000000 ) ) ;
#26097=DIRECTION ( 'NONE',  ( -1.000000000000000000, 0.000000000000000000, 0.000000000000000000 ) ) ;
#26100=ORIENTED_EDGE ( 'NONE', *, *, #21789, .F. ) ;
#26102=CARTESIAN_POINT ( 'NONE',  ( 117.5000000000000000, 182.4348187808683690, 102.3881375866409513 ) ) ;
#26118=FACE_OUTER_BOUND ( 'NONE', #7869, .T. ) ;
#26130=CARTESIAN_POINT ( 'NONE',  ( 115.4999999999999858, 207.9999999999998010, -89.64869280115067340 ) ) ;
#26195=DIRECTION ( 'NONE',  ( -1.000000000000000000, -0.000000000000000000, -0.000000000000000000 ) ) ;
#26212=AXIS2_PLACEMENT_3D ( 'NONE', #22032, #15708, #28660 ) ;
#26253=EDGE_LOOP ( 'NONE', ( #17586, #31910, #454, #20621 ) ) ;
#26257=EDGE_CURVE ( 'NONE', #10430, #25798, #11180, .T. ) ;
#26258=EDGE_LOOP ( 'NONE', ( #16382, #15748 ) ) ;
#26291=AXIS2_PLACEMENT_3D ( 'NONE', #1831, #22611, #32998 ) ;
#26322=LINE ( 'NONE', #26981, #28242 ) ;
#26348=CARTESIAN_POINT ( 'NONE',  ( 77.50000000000000000, 155.0000000000000000, -6.938893903907228378E-15 ) ) ;
#26555=CIRCLE ( 'NONE', #28206, 2.149999999999985256 ) ;
#26575=VECTOR ( 'NONE', #12561, 1000.000000000000000 ) ;
#26579=EDGE_CURVE ( 'NONE', #13101, #20988, #15624, .T. ) ;
#26637=DIRECTION ( 'NONE',  ( 0.000000000000000000, 0.000000000000000000, 1.000000000000000000 ) ) ;
#26651=EDGE_CURVE ( 'NONE', #31059, #6774, #9624, .T. ) ;
#26669=ORIENTED_EDGE ( 'NONE', *, *, #12723, .T. ) ;
#26673=DIRECTION ( 'NONE',  ( -1.000000000000000000, 0.000000000000000000, 0.000000000000000000 ) ) ;
#26685=CARTESIAN_POINT ( 'NONE',  ( 72.99495483890930814, 155.0000000000000000, -6.938893903907228378E-15 ) ) ;
#26717=FILL_AREA_STYLE_COLOUR ( '', #4586 ) ;
#26718=CARTESIAN_POINT ( 'NONE',  ( 107.5000000000000000, 155.0000000000000000, -6.938893903907228378E-15 ) ) ;
#26785=DIRECTION ( 'NONE',  ( 0.000000000000000000, -0.7071067811865330288, 0.7071067811865621167 ) ) ;
#26812=CIRCLE ( 'NONE', #26291, 2.149999999999985256 ) ;
#26831=ORIENTED_EDGE ( 'NONE', *, *, #15906, .F. ) ;
#26881=LINE ( 'NONE', #24159, #8610 ) ;
#26883=AXIS2_PLACEMENT_3D ( 'NONE', #10084, #25570, #2234 ) ;
#26951=DIRECTION ( 'NONE',  ( 1.000000000000000000, 0.000000000000000000, 0.000000000000000000 ) ) ;
#26956=ORIENTED_EDGE ( 'NONE', *, *, #33465, .F. ) ;
#26981=CARTESIAN_POINT ( 'NONE',  ( 117.5000000000000000, 155.0000000000000000, 97.99999999999997158 ) ) ;
#27001=DIRECTION ( 'NONE',  ( 1.000000000000000000, 0.000000000000000000, 0.000000000000000000 ) ) ;
#27008=ORIENTED_EDGE ( 'NONE', *, *, #4398, .T. ) ;
#27025=CYLINDRICAL_SURFACE ( 'NONE', #29078, 2.149999999999999023 ) ;
#27089=EDGE_LOOP ( 'NONE', ( #25052, #28978 ) ) ;
#27095=PLANE ( 'NONE',  #971 ) ;
#27113=DIRECTION ( 'NONE',  ( 0.000000000000000000, -0.7071067811865540120, -0.7071067811865411334 ) ) ;
#27117=CARTESIAN_POINT ( 'NONE',  ( 67.50000000000000000, 155.0000000000000000, 13.49999999999996270 ) ) ;
#27123=AXIS2_PLACEMENT_3D ( 'NONE', #16651, #12222, #22610 ) ;
#27139=VERTEX_POINT ( 'NONE', #23759 ) ;
#27168=EDGE_LOOP ( 'NONE', ( #4902, #1268 ) ) ;
#27181=VERTEX_POINT ( 'NONE', #12869 ) ;
#27219=FACE_BOUND ( 'NONE', #27089, .T. ) ;
#27259=ORIENTED_EDGE ( 'NONE', *, *, #18036, .F. ) ;
#27275=EDGE_CURVE ( 'NONE', #5869, #4349, #24351, .T. ) ;
#27284=PRODUCT_DEFINITION ( 'UNKNOWN', '', #13194, #903 ) ;
#27295=EDGE_LOOP ( 'NONE', ( #24502, #17934 ) ) ;
#27347=CIRCLE ( 'NONE', #1788, 112.0000000000000426 ) ;
#27381=FACE_BOUND ( 'NONE', #7545, .T. ) ;
#27392=CARTESIAN_POINT ( 'NONE',  ( 115.4999999999999858, 155.0000000000000000, -6.938893903907228378E-15 ) ) ;
#27469=ORIENTED_EDGE ( 'NONE', *, *, #11204, .F. ) ;
#27490=CARTESIAN_POINT ( 'NONE',  ( 117.5000000000000000, 155.0000000000000000, -98.00000000000000000 ) ) ;
#27512=ORIENTED_EDGE ( 'NONE', *, *, #22865, .T. ) ;
#27582=ORIENTED_EDGE ( 'NONE', *, *, #2287, .F. ) ;
#27592=CIRCLE ( 'NONE', #21088, 7.500000000000015099 ) ;
#27622=AXIS2_PLACEMENT_3D ( 'NONE', #32874, #27760, #28102 ) ;
#27624=ORIENTED_EDGE ( 'NONE', *, *, #31268, .T. ) ;
#27633=EDGE_LOOP ( 'NONE', ( #5962, #7752, #29525, #32602 ) ) ;
#27652=DIRECTION ( 'NONE',  ( -1.000000000000000000, -0.000000000000000000, 0.000000000000000000 ) ) ;
#27666=ORIENTED_EDGE ( 'NONE', *, *, #11894, .T. ) ;
#27679=EDGE_LOOP ( 'NONE', ( #32657, #33219, #862, #13367 ) ) ;
#27717=CARTESIAN_POINT ( 'NONE',  ( 67.50000000000000000, 155.0000000000000000, -6.938893903907228378E-15 ) ) ;
#27727=FACE_OUTER_BOUND ( 'NONE', #4426, .T. ) ;
#27744=DIRECTION ( 'NONE',  ( 0.000000000000000000, 0.000000000000000000, 1.000000000000000000 ) ) ;
#27760=DIRECTION ( 'NONE',  ( 0.000000000000000000, 1.000000000000000000, -1.224646799147353207E-16 ) ) ;
#27762=VERTEX_POINT ( 'NONE', #17265 ) ;
#27788=DIRECTION ( 'NONE',  ( -1.000000000000000000, -0.000000000000000000, -0.000000000000000000 ) ) ;
#27838=EDGE_CURVE ( 'NONE', #28486, #31748, #18906, .T. ) ;
#27886=LINE ( 'NONE', #18015, #26575 ) ;
#27911=AXIS2_PLACEMENT_3D ( 'NONE', #23413, #77, #15736 ) ;
#27915=CARTESIAN_POINT ( 'NONE',  ( 77.50000000000000000, 155.0000000000000000, -6.938893903907228378E-15 ) ) ;
#27936=CIRCLE ( 'NONE', #8893, 2.149999999999984812 ) ;
#27976=CARTESIAN_POINT ( 'NONE',  ( 79.50000000000000000, 155.0000000000000000, -6.938893903907228378E-15 ) ) ;
#27979=CARTESIAN_POINT ( 'NONE',  ( 117.5000000000000000, 102.0000000000001990, 91.79869280115065067 ) ) ;
#27995=CARTESIAN_POINT ( 'NONE',  ( 115.4999999999999858, 127.5651812191323557, -102.3881375866411645 ) ) ;
#28006=CARTESIAN_POINT ( 'NONE',  ( 115.4999999999999858, 183.9550983604194698, 103.9084171661920095 ) ) ;
#28090=ORIENTED_EDGE ( 'NONE', *, *, #22842, .T. ) ;
#28098=CLOSED_SHELL ( 'NONE', ( #20604, #33318, #10618, #22898, #7540, #3354, #2516, #13083, #14768, #11831, #14519, #10847, #9016, #14968, #2808, #30158, #14316, #24089, #33560, #24681, #29361, #12254, #19553, #28976, #4332, #18469, #30211, #9100, #25824, #1798, #7427, #7254, #13469, #18136, #20649, #11637, #6592, #6245, #7190, #20587 ) ) ;
#28102=DIRECTION ( 'NONE',  ( 0.000000000000000000, 0.000000000000000000, 1.000000000000000000 ) ) ;
#28106=CARTESIAN_POINT ( 'NONE',  ( 115.4999999999999858, 248.9486928011511679, 52.99999999999880629 ) ) ;
#28119=AXIS2_PLACEMENT_3D ( 'NONE', #19371, #9486, #12041 ) ;
#28138=EDGE_CURVE ( 'NONE', #21331, #33564, #31723, .T. ) ;
#28142=LINE ( 'NONE', #30877, #15587 ) ;
#28165=CARTESIAN_POINT ( 'NONE',  ( 117.5000000000000000, 257.3881375866408803, -27.43481878086871717 ) ) ;
#28206=AXIS2_PLACEMENT_3D ( 'NONE', #23974, #8638, #29593 ) ;
#28241=CARTESIAN_POINT ( 'NONE',  ( 117.5000000000000000, 155.0000000000000000, -112.0000000000000426 ) ) ;
#28242=VECTOR ( 'NONE', #18991, 1000.000000000000000 ) ;
#28247=DIRECTION ( 'NONE',  ( 0.000000000000000000, 0.7071067811865434649, -0.7071067811865515695 ) ) ;
#28263=DIRECTION ( 'NONE',  ( 0.000000000000000000, 0.000000000000000000, -1.000000000000000000 ) ) ;
#28279=VERTEX_POINT ( 'NONE', #22167 ) ;
#28317=CARTESIAN_POINT ( 'NONE',  ( 115.4999999999999858, 102.0000000000001990, 91.79869280115065067 ) ) ;
#28332=DIRECTION ( 'NONE',  ( 0.000000000000000000, 0.000000000000000000, 1.000000000000000000 ) ) ;
#28340=CARTESIAN_POINT ( 'NONE',  ( 117.5000000000000000, 155.0000000000000000, 99.99999999999997158 ) ) ;
#28351=ORIENTED_EDGE ( 'NONE', *, *, #2287, .T. ) ;
#28374=CARTESIAN_POINT ( 'NONE',  ( 115.4999999999999858, 54.13214199290997897, 25.91453920131689870 ) ) ;
#28383=CARTESIAN_POINT ( 'NONE',  ( 79.50000000000000000, 155.0000000000000000, 69.99999999999998579 ) ) ;
#28408=CIRCLE ( 'NONE', #14237, 15.50000000000001066 ) ;
#28438=AXIS2_PLACEMENT_3D ( 'NONE', #23857, #8364, #5787 ) ;
#28461=DIRECTION ( 'NONE',  ( 0.000000000000000000, 0.000000000000000000, -1.000000000000000000 ) ) ;
#28486=VERTEX_POINT ( 'NONE', #15008 ) ;
#28494=ORIENTED_EDGE ( 'NONE', *, *, #21554, .T. ) ;
#28503=CIRCLE ( 'NONE', #2383, 2.150000000000004352 ) ;
#28511=AXIS2_PLACEMENT_3D ( 'NONE', #23560, #230, #10624 ) ;
#28534=EDGE_CURVE ( 'NONE', #10769, #7638, #2907, .T. ) ;
#28546=DIRECTION ( 'NONE',  ( 1.000000000000000000, -0.000000000000000000, -0.000000000000000000 ) ) ;
#28550=DIRECTION ( 'NONE',  ( 0.000000000000000000, 0.000000000000000000, -1.000000000000000000 ) ) ;
#28660=DIRECTION ( 'NONE',  ( 0.000000000000000000, 0.000000000000000000, -1.000000000000000000 ) ) ;
#28699=CARTESIAN_POINT ( 'NONE',  ( 117.5000000000000000, 182.4348187808683690, 102.3881375866409513 ) ) ;
#28714=AXIS2_PLACEMENT_3D ( 'NONE', #13169, #23563, #15886 ) ;
#28760=CARTESIAN_POINT ( 'NONE',  ( 115.4999999999999858, 207.9999999999998010, -91.79869280115066488 ) ) ;
#28763=DIRECTION ( 'NONE',  ( -1.000000000000000000, 0.000000000000000000, -0.000000000000000000 ) ) ;
#28792=SURFACE_STYLE_USAGE ( .BOTH. , #8180 ) ;
#28793=DIRECTION ( 'NONE',  ( 0.000000000000000000, -0.7071067811865330288, 0.7071067811865621167 ) ) ;
#28821=DIRECTION ( 'NONE',  ( 0.000000000000000000, 0.7071067811865540120, 0.7071067811865411334 ) ) ;
#28856=EDGE_LOOP ( 'NONE', ( #20841, #9487 ) ) ;
#28873=CIRCLE ( 'NONE', #33235, 100.0000000000000000 ) ;
#28904=EDGE_CURVE ( 'NONE', #5683, #10401, #25452, .T. ) ;
#28907=PRESENTATION_STYLE_ASSIGNMENT (( #462 ) ) ;
#28976=ADVANCED_FACE ( 'NONE', ( #22809 ), #14631, .F. ) ;
#28978=ORIENTED_EDGE ( 'NONE', *, *, #2624, .F. ) ;
#28984=DIRECTION ( 'NONE',  ( 0.000000000000000000, 0.000000000000000000, -1.000000000000000000 ) ) ;
#28988=AXIS2_PLACEMENT_3D ( 'NONE', #9792, #17451, #4000 ) ;
#28993=CYLINDRICAL_SURFACE ( 'NONE', #20815, 112.0000000000000426 ) ;
#29010=VECTOR ( 'NONE', #15548, 1000.000000000000000 ) ;
#29042=DIRECTION ( 'NONE',  ( 0.000000000000000000, 0.000000000000000000, -1.000000000000000000 ) ) ;
#29072=UNCERTAINTY_MEASURE_WITH_UNIT (LENGTH_MEASURE( 1.000000000000000082E-05 ), #16114, 'distance_accuracy_value', 'NONE');
#29076=DIRECTION ( 'NONE',  ( 1.000000000000000000, 0.000000000000000000, 0.000000000000000000 ) ) ;
#29078=AXIS2_PLACEMENT_3D ( 'NONE', #304, #10703, #4362 ) ;
#29167=DIRECTION ( 'NONE',  ( -1.000000000000000000, -0.000000000000000000, -0.000000000000000000 ) ) ;
#29173=EDGE_CURVE ( 'NONE', #28486, #33027, #23148, .T. ) ;
#29187=EDGE_LOOP ( 'NONE', ( #21343, #21591, #4649, #17971 ) ) ;
#29206=AXIS2_PLACEMENT_3D ( 'NONE', #20938, #31330, #5916 ) ;
#29274=DIRECTION ( 'NONE',  ( -1.000000000000000000, -0.000000000000000000, 0.000000000000000000 ) ) ;
#29289=VECTOR ( 'NONE', #28763, 1000.000000000000000 ) ;
#29361=ADVANCED_FACE ( 'NONE', ( #17694, #25871, #15805, #2198, #2537, #307, #7317, #20753, #12920, #22973 ), #33372, .T. ) ;
#29368=DIRECTION ( 'NONE',  ( 0.000000000000000000, 0.7071067811865540120, 0.7071067811865411334 ) ) ;
#29372=EDGE_CURVE ( 'NONE', #15657, #6774, #26555, .T. ) ;
#29432=CIRCLE ( 'NONE', #75, 7.500000000000015099 ) ;
#29438=DIRECTION ( 'NONE',  ( 0.000000000000000000, 0.7071067811865506814, 0.7071067811865442421 ) ) ;
#29500=CYLINDRICAL_SURFACE ( 'NONE', #6621, 97.99999999999997158 ) ;
#29525=ORIENTED_EDGE ( 'NONE', *, *, #4948, .T. ) ;
#29556=VECTOR ( 'NONE', #2145, 1000.000000000000000 ) ;
#29588=DIRECTION ( 'NONE',  ( -1.000000000000000000, 0.000000000000000000, 0.000000000000000000 ) ) ;
#29593=DIRECTION ( 'NONE',  ( 0.000000000000000000, 0.000000000000000000, 1.000000000000000000 ) ) ;
#29606=EDGE_LOOP ( 'NONE', ( #20255, #23744 ) ) ;
#29622=CARTESIAN_POINT ( 'NONE',  ( 117.5000000000000000, 155.0000000000000000, -98.00000000000000000 ) ) ;
#29700=CARTESIAN_POINT ( 'NONE',  ( 115.4999999999999858, 180.9145392013172682, 100.8678580070898931 ) ) ;
#29711=FACE_OUTER_BOUND ( 'NONE', #2811, .T. ) ;
#29807=AXIS2_PLACEMENT_3D ( 'NONE', #24691, #1852, #32679 ) ;
#29875=CIRCLE ( 'NONE', #21767, 2.149999999999974598 ) ;
#29895=AXIS2_PLACEMENT_3D ( 'NONE', #8559, #5670, #15891 ) ;
#29905=ORIENTED_EDGE ( 'NONE', *, *, #14985, .F. ) ;
#29927=LINE ( 'NONE', #6580, #9354 ) ;
#29958=DIRECTION ( 'NONE',  ( 1.000000000000000000, 0.000000000000000000, 0.000000000000000000 ) ) ;
#30017=VERTEX_POINT ( 'NONE', #19451 ) ;
#30034=ORIENTED_EDGE ( 'NONE', *, *, #26651, .T. ) ;
#30084=CARTESIAN_POINT ( 'NONE',  ( 77.50000000000000000, 155.0000000000000000, -6.938893903907228378E-15 ) ) ;
#30137=CARTESIAN_POINT ( 'NONE',  ( 77.50000000000000000, 155.0000000000000000, -6.938893903907228378E-15 ) ) ;
#30158=ADVANCED_FACE ( 'NONE', ( #13371 ), #15188, .T. ) ;
#30179=DIRECTION ( 'NONE',  ( 1.000000000000000000, 0.000000000000000000, 0.000000000000000000 ) ) ;
#30205=DIRECTION ( 'NONE',  ( -1.000000000000000000, 0.000000000000000000, 0.000000000000000000 ) ) ;
#30211=ADVANCED_FACE ( 'NONE', ( #12463 ), #7024, .F. ) ;
#30230=DIRECTION ( 'NONE',  ( -1.000000000000000000, 0.000000000000000000, 0.000000000000000000 ) ) ;
#30327=AXIS2_PLACEMENT_3D ( 'NONE', #2336, #14938, #30786 ) ;
#30364=COLOUR_RGB ( '', 0.72549020, 0.75294118, 0.79215686) ;
#30392=DIRECTION ( 'NONE',  ( -1.000000000000000000, 0.000000000000000000, 0.000000000000000000 ) ) ;
#30417=FACE_BOUND ( 'NONE', #13502, .T. ) ;
#30420=VERTEX_POINT ( 'NONE', #18251 ) ;
#30480=CARTESIAN_POINT ( 'NONE',  ( 117.5000000000000000, 155.0000000000000000, -6.938893903907228378E-15 ) ) ;
#30542=ORIENTED_EDGE ( 'NONE', *, *, #4964, .T. ) ;
#30624=VERTEX_POINT ( 'NONE', #23355 ) ;
#30630=SURFACE_STYLE_FILL_AREA ( #20229 ) ;
#30645=CIRCLE ( 'NONE', #5080, 2.149999999999994138 ) ;
#30654=DIRECTION ( 'NONE',  ( 1.000000000000000000, 0.000000000000000000, 0.000000000000000000 ) ) ;
#30683=LINE ( 'NONE', #6657, #32561 ) ;
#30716=ORIENTED_EDGE ( 'NONE', *, *, #14160, .F. ) ;
#30731=CARTESIAN_POINT ( 'NONE',  ( 115.4999999999999858, 126.0449016395812691, -103.9084171661922227 ) ) ;
#30786=DIRECTION ( 'NONE',  ( 0.000000000000000000, 0.000000000000000000, 1.000000000000000000 ) ) ;
#30830=AXIS2_PLACEMENT_3D ( 'NONE', #28317, #26097, #4637 ) ;
#30859=VECTOR ( 'NONE', #7072, 1000.000000000000000 ) ;
#30877=CARTESIAN_POINT ( 'NONE',  ( 72.99495483890930814, 155.0000000000000000, 15.50000000000000355 ) ) ;
#30964=ORIENTED_EDGE ( 'NONE', *, *, #14300, .T. ) ;
#30975=AXIS2_PLACEMENT_3D ( 'NONE', #13870, #3150, #24436 ) ;
#30980=CARTESIAN_POINT ( 'NONE',  ( 115.4999999999999858, 129.0854607986834139, -100.8678580070901063 ) ) ;
#30992=CARTESIAN_POINT ( 'NONE',  ( 115.4999999999999858, 255.8678580070898363, -25.91453920131763056 ) ) ;
#31016=ORIENTED_EDGE ( 'NONE', *, *, #17916, .F. ) ;
#31026=CARTESIAN_POINT ( 'NONE',  ( 79.50000000000000000, 155.0000000000000000, -6.938893903907228378E-15 ) ) ;
#31059=VERTEX_POINT ( 'NONE', #15039 ) ;
#31061=DIRECTION ( 'NONE',  ( -1.000000000000000000, -0.000000000000000000, -0.000000000000000000 ) ) ;
#31063=AXIS2_PLACEMENT_3D ( 'NONE', #26718, #19057, #833 ) ;
#31147=CYLINDRICAL_SURFACE ( 'NONE', #17628, 2.149999999999999023 ) ;
#31166=VERTEX_POINT ( 'NONE', #21945 ) ;
#31193=CARTESIAN_POINT ( 'NONE',  ( 115.4999999999999858, 52.61186241335891367, 27.43481878086798176 ) ) ;
#31210=EDGE_CURVE ( 'NONE', #21928, #24566, #18851, .T. ) ;
#31245=LINE ( 'NONE', #18288, #32049 ) ;
#31268=EDGE_CURVE ( 'NONE', #21649, #17667, #19226, .T. ) ;
#31270=DIRECTION ( 'NONE',  ( 1.000000000000000000, 0.000000000000000000, 0.000000000000000000 ) ) ;
#31287=DIRECTION ( 'NONE',  ( 0.000000000000000000, 0.000000000000000000, 1.000000000000000000 ) ) ;
#31298=DIRECTION ( 'NONE',  ( 0.000000000000000000, 0.000000000000000000, 1.000000000000000000 ) ) ;
#31330=DIRECTION ( 'NONE',  ( -1.000000000000000000, 0.000000000000000000, 0.000000000000000000 ) ) ;
#31339=CARTESIAN_POINT ( 'NONE',  ( 77.50000000000000000, 155.0000000000000000, -6.938893903907228378E-15 ) ) ;
#31384=EDGE_LOOP ( 'NONE', ( #22747, #20096, #15540, #31499 ) ) ;
#31450=DIRECTION ( 'NONE',  ( 0.000000000000000000, 0.000000000000000000, -1.000000000000000000 ) ) ;
#31473=CARTESIAN_POINT ( 'NONE',  ( 107.5000000000000000, 155.0000000000000000, -6.938893903907228378E-15 ) ) ;
#31499=ORIENTED_EDGE ( 'NONE', *, *, #5023, .T. ) ;
#31532=ORIENTED_EDGE ( 'NONE', *, *, #6031, .T. ) ;
#31537=CARTESIAN_POINT ( 'NONE',  ( 115.4999999999999858, 102.0000000000001990, 93.94869280115064214 ) ) ;
#31545=VECTOR ( 'NONE', #21792, 1000.000000000000000 ) ;
#31573=ORIENTED_EDGE ( 'NONE', *, *, #13514, .T. ) ;
#31582=CARTESIAN_POINT ( 'NONE',  ( 107.5000000000000000, 155.0000000000000000, -6.938893903907228378E-15 ) ) ;
#31625=DIRECTION ( 'NONE',  ( 0.000000000000000000, 1.000000000000000000, -9.682177540335733218E-15 ) ) ;
#31639=DIRECTION ( 'NONE',  ( 0.000000000000000000, 0.000000000000000000, -1.000000000000000000 ) ) ;
#31655=VERTEX_POINT ( 'NONE', #10369 ) ;
#31681=DIRECTION ( 'NONE',  ( -1.000000000000000000, -0.000000000000000000, 0.000000000000000000 ) ) ;
#31723=LINE ( 'NONE', #11450, #24916 ) ;
#31747=DIRECTION ( 'NONE',  ( 1.000000000000000000, 0.000000000000000000, 0.000000000000000000 ) ) ;
#31748=VERTEX_POINT ( 'NONE', #23636 ) ;
#31761=AXIS2_PLACEMENT_3D ( 'NONE', #18807, #19311, #32251 ) ;
#31823=FACE_OUTER_BOUND ( 'NONE', #26253, .T. ) ;
#31896=ORIENTED_EDGE ( 'NONE', *, *, #3252, .F. ) ;
#31910=ORIENTED_EDGE ( 'NONE', *, *, #32890, .T. ) ;
#31929=FACE_OUTER_BOUND ( 'NONE', #32196, .T. ) ;
#31930=AXIS2_PLACEMENT_3D ( 'NONE', #4688, #28546, #10326 ) ;
#31991=CARTESIAN_POINT ( 'NONE',  ( 115.4999999999999858, 127.5651812191323557, -102.3881375866411645 ) ) ;
#31998=ORIENTED_EDGE ( 'NONE', *, *, #25399, .F. ) ;
#32000=SHAPE_REPRESENTATION_RELATIONSHIP ( 'NONE' , 'NONE' ,  #19592, #16530 ) ;
#32044=ORIENTED_EDGE ( 'NONE', *, *, #22865, .F. ) ;
#32049=VECTOR ( 'NONE', #5338, 1000.000000000000000 ) ;
#32070=CARTESIAN_POINT ( 'NONE',  ( 115.4999999999999858, 248.9486928011511679, 52.99999999999880629 ) ) ;
#32077=ORIENTED_EDGE ( 'NONE', *, *, #23883, .F. ) ;
#32196=EDGE_LOOP ( 'NONE', ( #25581, #2472, #15821, #27259 ) ) ;
#32251=DIRECTION ( 'NONE',  ( 0.000000000000000000, 0.000000000000000000, 1.000000000000000000 ) ) ;
#32254=VECTOR ( 'NONE', #10622, 1000.000000000000000 ) ;
#32264=DIRECTION ( 'NONE',  ( -1.000000000000000000, 0.000000000000000000, 0.000000000000000000 ) ) ;
#32282=VERTEX_POINT ( 'NONE', #5781 ) ;
#32283=FACE_OUTER_BOUND ( 'NONE', #19548, .T. ) ;
#32284=CIRCLE ( 'NONE', #5639, 13.50000000000001066 ) ;
#32303=DIRECTION ( 'NONE',  ( 0.000000000000000000, 0.000000000000000000, -1.000000000000000000 ) ) ;
#32386=CARTESIAN_POINT ( 'NONE',  ( 77.50000000000000000, 155.0000000000000000, -15.50000000000001776 ) ) ;
#32410=DIRECTION ( 'NONE',  ( 0.000000000000000000, 0.7071067811865434649, -0.7071067811865515695 ) ) ;
#32411=ORIENTED_EDGE ( 'NONE', *, *, #15353, .T. ) ;
#32429=CYLINDRICAL_SURFACE ( 'NONE', #16264, 7.500000000000015099 ) ;
#32451=EDGE_LOOP ( 'NONE', ( #6217, #21387, #24665, #4930 ) ) ;
#32481=AXIS2_PLACEMENT_3D ( 'NONE', #15945, #2686, #31298 ) ;
#32561=VECTOR ( 'NONE', #20110, 1000.000000000000000 ) ;
#32565=ORIENTED_EDGE ( 'NONE', *, *, #25125, .F. ) ;
#32579=AXIS2_PLACEMENT_3D ( 'NONE', #9953, #25617, #2283 ) ;
#32582=CYLINDRICAL_SURFACE ( 'NONE', #3182, 2.149999999999996803 ) ;
#32602=ORIENTED_EDGE ( 'NONE', *, *, #33299, .F. ) ;
#32618=CARTESIAN_POINT ( 'NONE',  ( 79.50000000000000000, 155.0000000000000000, -6.938893903907228378E-15 ) ) ;
#32619=ORIENTED_EDGE ( 'NONE', *, *, #13553, .T. ) ;
#32636=DIRECTION ( 'NONE',  ( 0.000000000000000000, 0.000000000000000000, 1.000000000000000000 ) ) ;
#32654=EDGE_LOOP ( 'NONE', ( #10525, #414, #15695, #28494 ) ) ;
#32657=ORIENTED_EDGE ( 'NONE', *, *, #26000, .F. ) ;
#32666=CARTESIAN_POINT ( 'NONE',  ( 115.4999999999999858, 155.0000000000000000, 112.0000000000000426 ) ) ;
#32679=DIRECTION ( 'NONE',  ( 0.000000000000000000, 0.000000000000000000, -1.000000000000000000 ) ) ;
#32736=AXIS2_PLACEMENT_3D ( 'NONE', #3937, #30179, #12454 ) ;
#32741=DIRECTION ( 'NONE',  ( -1.000000000000000000, -0.000000000000000000, -0.000000000000000000 ) ) ;
#32827=EDGE_LOOP ( 'NONE', ( #6531, #27666, #13757, #4802 ) ) ;
#32830=FACE_BOUND ( 'NONE', #26258, .T. ) ;
#32874=CARTESIAN_POINT ( 'NONE',  ( 107.5000000000000000, 155.0000000000000000, 69.99999999999998579 ) ) ;
#32890=EDGE_CURVE ( 'NONE', #24566, #21928, #28503, .T. ) ;
#32961=ORIENTED_EDGE ( 'NONE', *, *, #4490, .F. ) ;
#32989=ORIENTED_EDGE ( 'NONE', *, *, #3894, .F. ) ;
#32998=DIRECTION ( 'NONE',  ( 0.000000000000000000, 0.000000000000000000, -1.000000000000000000 ) ) ;
#33006=CARTESIAN_POINT ( 'NONE',  ( 117.5000000000000000, 65.35130719884917028, -52.99999999999947420 ) ) ;
#33027=VERTEX_POINT ( 'NONE', #4690 ) ;
#33036=VERTEX_POINT ( 'NONE', #4352 ) ;
#33172=ORIENTED_EDGE ( 'NONE', *, *, #5953, .T. ) ;
#33192=DIRECTION ( 'NONE',  ( -1.000000000000000000, 0.000000000000000000, -0.000000000000000000 ) ) ;
#33219=ORIENTED_EDGE ( 'NONE', *, *, #21235, .F. ) ;
#33235=AXIS2_PLACEMENT_3D ( 'NONE', #187, #13126, #23682 ) ;
#33261=ORIENTED_EDGE ( 'NONE', *, *, #28534, .T. ) ;
#33299=EDGE_CURVE ( 'NONE', #12934, #13672, #4862, .T. ) ;
#33318=ADVANCED_FACE ( 'NONE', ( #15421 ), #2481, .F. ) ;
#33343=CIRCLE ( 'NONE', #14283, 2.149999999999985256 ) ;
#33360=LINE ( 'NONE', #22962, #13122 ) ;
#33372=PLANE ( 'NONE',  #9150 ) ;
#33396=DIRECTION ( 'NONE',  ( 1.000000000000000000, 0.000000000000000000, 0.000000000000000000 ) ) ;
#33431=( GEOMETRIC_REPRESENTATION_CONTEXT ( 3 ) GLOBAL_UNCERTAINTY_ASSIGNED_CONTEXT ( ( #22633 ) ) GLOBAL_UNIT_ASSIGNED_CONTEXT ( ( #506, #21277, #10573 ) ) REPRESENTATION_CONTEXT ( 'NONE', 'WORKASPACE' ) );
#33449=CARTESIAN_POINT ( 'NONE',  ( 115.4999999999999858, 127.5651812191323557, -102.3881375866411645 ) ) ;
#33465=EDGE_CURVE ( 'NONE', #30017, #30624, #24695, .T. ) ;
#33511=EDGE_CURVE ( 'NONE', #31655, #17667, #10023, .T. ) ;
#33560=ADVANCED_FACE ( 'NONE', ( #3299 ), #11481, .T. ) ;
#33564=VERTEX_POINT ( 'NONE', #29700 ) ;
#33566=DIRECTION ( 'NONE',  ( -1.000000000000000000, 0.000000000000000000, -0.000000000000000000 ) ) ;
#33615=LINE ( 'NONE', #28340, #32254 ) ;
#33649=CARTESIAN_POINT ( 'NONE',  ( 115.4999999999999858, 63.20130719884917170, -52.99999999999946709 ) ) ;
ENDSEC;
END-ISO-10303-21;
